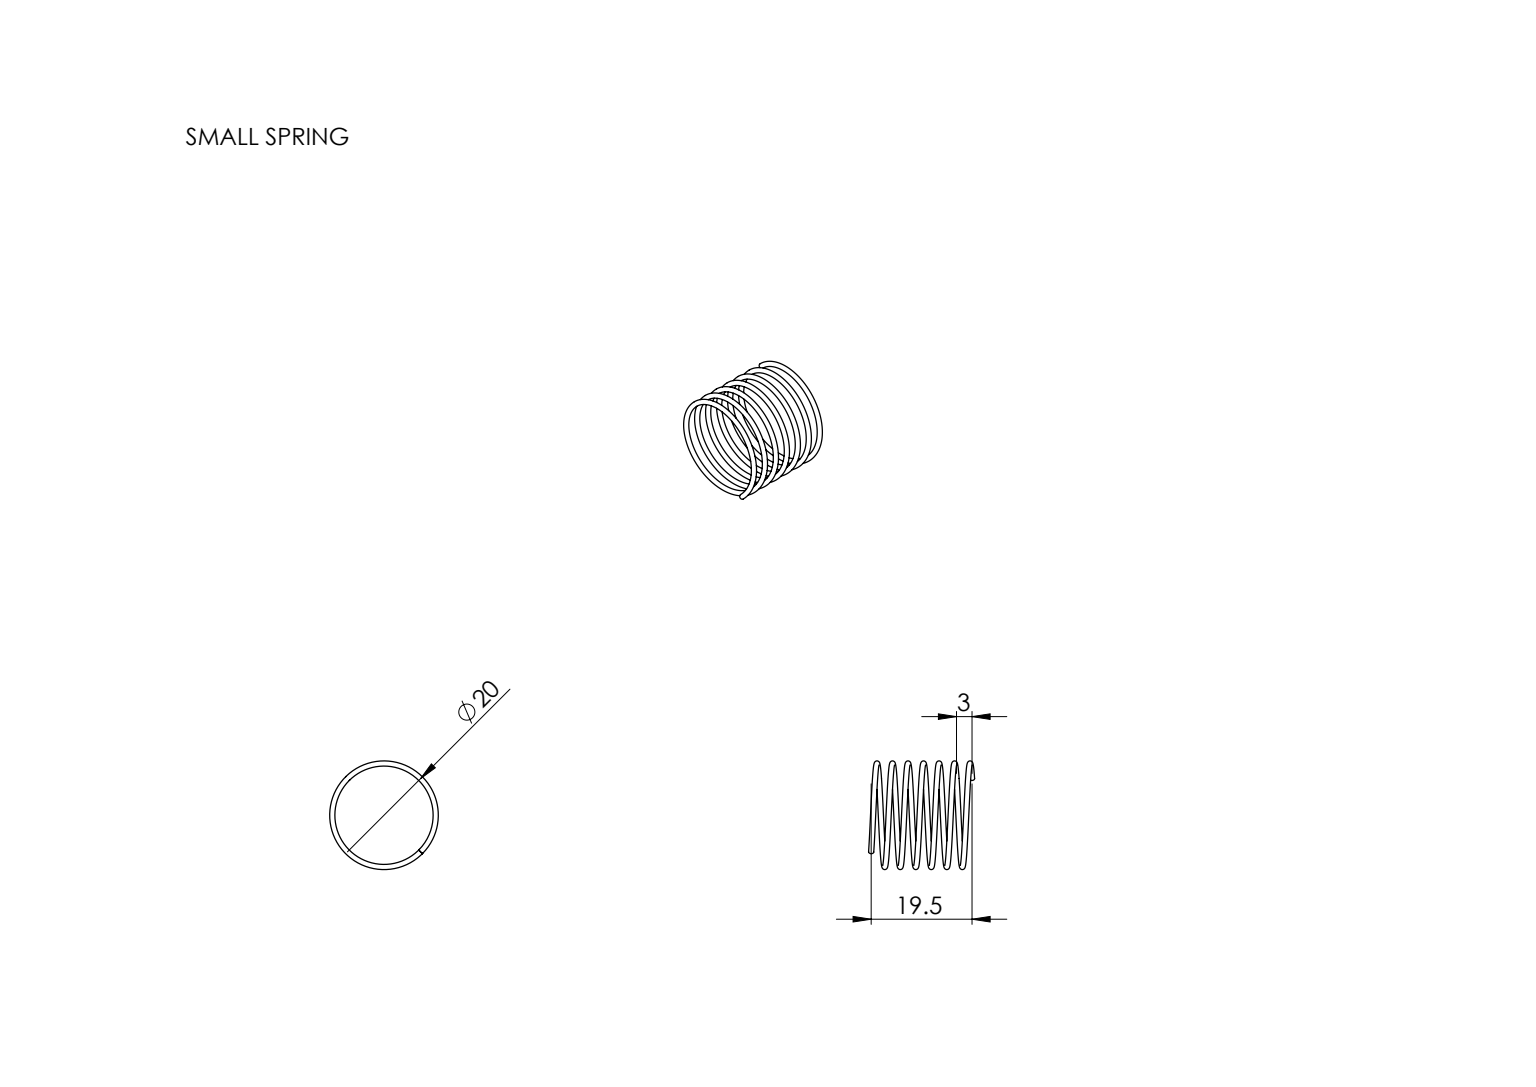
ISO-10303-21;
HEADER;
FILE_DESCRIPTION (('STEP AP214'),
    '1' );
FILE_NAME ('small spring.step',
    '2026-10-08T13:22:57',
    ( '' ),
    ( '' ),
    'SwSTEP 2.0',
    'SolidWorks 2026',
    '' );
FILE_SCHEMA (( 'AUTOMOTIVE_DESIGN' ));
ENDSEC;

DATA;
#1=CARTESIAN_POINT ( 'NONE',  ( -9.837026868206070418, 5.012215536711416952, 5.849999999999989875 ) ) ;
#6=CARTESIAN_POINT ( 'NONE',  ( 9.377220287599001836, 4.724406229267489543, 5.901137918078571687 ) ) ;
#7=CARTESIAN_POINT ( 'NONE',  ( 8.486213763410640709, 4.270415729527937465, 17.90113791807857524 ) ) ;
#23=CARTESIAN_POINT ( 'NONE',  ( -4.312909747525649706, -8.464561979789507973, 14.10000000000000142 ) ) ;
#24=CARTESIAN_POINT ( 'NONE',  ( 4.534861676072320158, -8.900167166472098046, 4.650000000000026112 ) ) ;
#34=CARTESIAN_POINT ( 'NONE',  ( -7.458344646081709328, 7.390897758835804687, 9.998862081921425116 ) ) ;
#40=CARTESIAN_POINT ( 'NONE',  ( -9.865911304835474738, -1.562606840307925848, 8.549999999999963407 ) ) ;
#41=CARTESIAN_POINT ( 'NONE',  ( 5.012215536711511987, -9.837026868205999364, 13.65000000000003233 ) ) ;
#50=CARTESIAN_POINT ( 'NONE',  ( 10.90442828429183919, 1.727091770866679532, 1.049999999999966738 ) ) ;
#55=CARTESIAN_POINT ( 'NONE',  ( 4.766900247265192903, 9.355568503977902850, 12.59999999999999964 ) ) ;
#60=CARTESIAN_POINT ( 'NONE',  ( 4.809394265263009061, 9.333916720356739916, 8.601137918078563871 ) ) ;
#61=CARTESIAN_POINT ( 'NONE',  ( -9.873755945037078874, -1.513077731353019706, 10.55113791807857204 ) ) ;
#72=CARTESIAN_POINT ( 'NONE',  ( 9.865911304835474738, 1.562606840307950051, 19.04999999999997939 ) ) ;
#73=CARTESIAN_POINT ( 'NONE',  ( 8.900167166472154889, -4.534861676072210912, 7.350000000000000533 ) ) ;
#83=CARTESIAN_POINT ( 'NONE',  ( 4.724406229267374968, 9.377220287599055126, 13.59886208192140167 ) ) ;
#84=CARTESIAN_POINT ( 'NONE',  ( 5.056896391392317724, -9.814260835640977731, 14.64886208192141659 ) ) ;
#90=CARTESIAN_POINT ( 'NONE',  ( -1.486127417882243895, 9.383039235653816590, 15.29999999999997939 ) ) ;
#91=CARTESIAN_POINT ( 'NONE',  ( 1.727091770866550968, 10.90442828429186761, 18.44999999999999218 ) ) ;
#99=CARTESIAN_POINT ( 'NONE',  ( -7.806708723663830618, -7.806708723663906113, 8.250000000000028422 ) ) ;
#102=( LENGTH_UNIT ( ) NAMED_UNIT ( * ) SI_UNIT ( .MILLI., .METRE. ) );
#105=CARTESIAN_POINT ( 'NONE',  ( -5.012215536711508435, 9.837026868206029562, 9.150000000000002132 ) ) ;
#108=CARTESIAN_POINT ( 'NONE',  ( -10.91227292449344155, -1.677562661911748965, 4.551137918078585365 ) ) ;
#109=CARTESIAN_POINT ( 'NONE',  ( 9.375578539472099848, -1.533232399699987702, 15.20113791807854575 ) ) ;
#121=CARTESIAN_POINT ( 'NONE',  ( 1.562606840307832368, 9.865911304835503159, 18.44999999999999218 ) ) ;
#122=CARTESIAN_POINT ( 'NONE',  ( 7.063212654743467489, 7.063212654743559860, 3.749999999999997335 ) ) ;
#125=CARTESIAN_POINT ( 'NONE',  ( 7.063212654743468377, 7.063212654743558083, 0.7499999999999762412 ) ) ;
#134=CARTESIAN_POINT ( 'NONE',  ( -8.442910196168309511, -4.355403765523546689, 6.398862081921404155 ) ) ;
#135=CARTESIAN_POINT ( 'NONE',  ( -5.056896391392315948, 9.814260835640997271, 16.14886208192145389 ) ) ;
#141=CARTESIAN_POINT ( 'NONE',  ( 1.562606840307832146, 9.865911304835508489, 15.44999999999997797 ) ) ;
#142=CARTESIAN_POINT ( 'NONE',  ( -9.333916720356675967, -4.809394265263095214, 12.39886208192140948 ) ) ;
#150=CARTESIAN_POINT ( 'NONE',  ( -4.766900247265192014, -9.355568503977867323, 8.099999999999996092 ) ) ;
#151=CARTESIAN_POINT ( 'NONE',  ( -4.766900247265192014, -9.355568503977867323, 8.099999999999996092 ) ) ;
#156=CARTESIAN_POINT ( 'NONE',  ( -5.012215536711508435, 9.837026868206020680, 18.15000000000000924 ) ) ;
#159=CARTESIAN_POINT ( 'NONE',  ( -4.967534682030703586, 9.859792900771061852, 17.15113791807853616 ) ) ;
#160=CARTESIAN_POINT ( 'NONE',  ( 4.490180821391514421, -8.922933199037132113, 12.65113791807859123 ) ) ;
#173=CARTESIAN_POINT ( 'NONE',  ( -1.439022436064386845, 9.390499931835535108, 8.301137918078554279 ) ) ;
#174=CARTESIAN_POINT ( 'NONE',  ( 1.486127417882244783, -9.383039235653782839, 7.800000000000029132 ) ) ;
#177=CARTESIAN_POINT ( 'NONE',  ( -4.312909747525649706, -8.464561979789507973, 2.099999999999990763 ) ) ;
#187=( NAMED_UNIT ( * ) PLANE_ANGLE_UNIT ( ) SI_UNIT ( $, .RADIAN. ) );
#190=CARTESIAN_POINT ( 'NONE',  ( -9.390499931835536884, 1.439022436064298249, 6.698862081921455491 ) ) ;
#191=CARTESIAN_POINT ( 'NONE',  ( -1.533232399700100057, 9.375578539472094519, 1.298862081921425604 ) ) ;
#199=CARTESIAN_POINT ( 'NONE',  ( -4.534861676072319270, 8.900167166472117586, 18.15000000000000924 ) ) ;
#200=CARTESIAN_POINT ( 'NONE',  ( -9.333916720356675967, -4.809394265263096990, 9.398862081921446787 ) ) ;
#206=MANIFOLD_SOLID_BREP ( 'Sweep1', #9455 ) ;
#209=CARTESIAN_POINT ( 'NONE',  ( -10.37072757624895836, 1.642561882922381145, 5.700000000000038369 ) ) ;
#210=CARTESIAN_POINT ( 'NONE',  ( 5.012215536711511987, -9.837026868205999364, 13.65000000000003233 ) ) ;
#213=CARTESIAN_POINT ( 'NONE',  ( 1.727091770866551412, 10.90442828429187117, 15.44999999999997797 ) ) ;
#216=CARTESIAN_POINT ( 'NONE',  ( 9.377220287599001836, 4.724406229267489543, 14.90113791807857879 ) ) ;
#217=CARTESIAN_POINT ( 'NONE',  ( -8.877401133907129704, 4.579542530753042406, 13.85113791807855321 ) ) ;
#226=CARTESIAN_POINT ( 'NONE',  ( 7.098671581784200768, 7.027753727702831021, 8.751137918078539357 ) ) ;
#227=CARTESIAN_POINT ( 'NONE',  ( -8.464561979789474222, -4.312909747525729642, 8.399999999999963052 ) ) ;
#238=( NAMED_UNIT ( * ) SI_UNIT ( $, .STERADIAN. ) SOLID_ANGLE_UNIT ( ) );
#240=CARTESIAN_POINT ( 'NONE',  ( 8.922933199037192509, -4.490180821391404287, 14.34886208192142831 ) ) ;
#242=CARTESIAN_POINT ( 'NONE',  ( -10.89658364409024749, -1.776620879821561694, 15.54886208192143293 ) ) ;
#245=CARTESIAN_POINT ( 'NONE',  ( 0.000000000000000000, 0.000000000000000000, 0.000000000000000000 ) ) ;
#249=CARTESIAN_POINT ( 'NONE',  ( 4.724406229267374968, 9.377220287599060455, 10.59886208192144075 ) ) ;
#258=CARTESIAN_POINT ( 'NONE',  ( 10.90442828429183919, 1.727091770866679532, 10.05000000000002736 ) ) ;
#259=CARTESIAN_POINT ( 'NONE',  ( -10.90442828429183919, -1.727091770866654663, 14.55000000000000249 ) ) ;
#263=CARTESIAN_POINT ( 'NONE',  ( -9.837026868206070418, 5.012215536711416952, 11.84999999999997478 ) ) ;
#266=CARTESIAN_POINT ( 'NONE',  ( 7.390897758835871301, -7.458344646081617846, 18.50113791807859087 ) ) ;
#267=CARTESIAN_POINT ( 'NONE',  ( 9.814260835641038128, -5.056896391392200485, 6.351137918078572753 ) ) ;
#272=CARTESIAN_POINT ( 'NONE',  ( -10.90442828429183919, -1.727091770866655329, 8.549999999999963407 ) ) ;
#278=CARTESIAN_POINT ( 'NONE',  ( 8.486213763410640709, 4.270415729527937465, 5.901137918078571687 ) ) ;
#279=CARTESIAN_POINT ( 'NONE',  ( -4.534861676072319270, 8.900167166472117586, 18.15000000000000924 ) ) ;
#292=CARTESIAN_POINT ( 'NONE',  ( -8.442910196168309511, -4.355403765523546689, 18.39886208192140771 ) ) ;
#293=CARTESIAN_POINT ( 'NONE',  ( 10.89658364409024749, 1.776620879821585897, 20.04886208192142050 ) ) ;
#300=CARTESIAN_POINT ( 'NONE',  ( 4.312909747525650594, 8.464561979789532842, 15.60000000000000320 ) ) ;
#301=CARTESIAN_POINT ( 'NONE',  ( 1.689666864740335894, -10.36326688006721497, 11.79886208192143471 ) ) ;
#307=CARTESIAN_POINT ( 'NONE',  ( 1.642561882922480621, -10.37072757624891750, 7.800000000000029132 ) ) ;
#316=CARTESIAN_POINT ( 'NONE',  ( -5.012215536711506658, 9.837026868206027785, 0.1499999999999952482 ) ) ;
#317=CARTESIAN_POINT ( 'NONE',  ( 7.842167650704563897, 7.771249796623202144, 8.751137918078539357 ) ) ;
#319=CARTESIAN_POINT ( 'NONE',  ( 1.727091770866550968, 10.90442828429187294, 3.450000000000006839 ) ) ;
#327=CARTESIAN_POINT ( 'NONE',  ( 8.877401133907127928, -4.579542530753017537, 9.351137918078563871 ) ) ;
#328=CARTESIAN_POINT ( 'NONE',  ( 8.464561979789474222, 4.312909747525755400, 18.90000000000002700 ) ) ;
#330=( BOUNDED_CURVE ( )  B_SPLINE_CURVE ( 2, ( #1514, #9215, #5487, #10036, #7667, #6246, #5333, #2234, #7861, #8431, #2948, #2187, #6092, #786, #3003, #6917, #1413, #3937, #8645, #6864, #4564, #3053, #741, #637, #9270, #3888, #10090, #7717, #2284, #1567, #6978, #5381, #8538, #4713, #7080, #3840, #3106, #6146, #10139, #1, #1463, #8488, #7032, #7766, #692, #1358, #583, #3729, #6197, #9372, #5429, #8589, #4663, #2129, #7814, #3158, #5271, #4512, #3992, #5682, #3258, #105, #8116, #4813, #4914, #7237, #6452, #5534, #6297, #8061, #7909, #3313, #4967, #989, #9631, #2434, #8693, #8897, #4042, #263, #9481, #942, #8852, #7290, #55, #6399, #1719, #4140, #3363, #3213, #7963, #836, #1045, #2534, #5579, #9576, #6498, #1811, #4190, #4763, #7340, #1665, #1762, #213, #7188, #894, #9677, #2480, #5634, #2585, #8800, #8742, #2384, #5730, #1614, #7138, #6349, #4864, #9527, #8010, #4087, #156, #8365, #9874, #1287, #9727, #9156, #7438, #2013, #5168, #7593 ),
 .UNSPECIFIED., .F., .T. ) 
 B_SPLINE_CURVE_WITH_KNOTS ( ( 3, 2, 2, 2, 2, 2, 2, 2, 2, 2, 2, 2, 2, 2, 2, 2, 2, 2, 2, 2, 2, 2, 2, 2, 2, 2, 2, 2, 2, 2, 2, 2, 2, 2, 2, 2, 2, 2, 2, 2, 2, 2, 2, 2, 2, 2, 2, 2, 2, 2, 2, 2, 2, 2, 2, 2, 2, 2, 2, 2, 2, 2, 2, 2, 2, 3 ),
 ( 0.000000000000000000, 0.01428571428571428527, 0.02857142857142857054, 0.04285714285714285060, 0.05714285714285714107, 0.07142857142857142461, 0.08571428571428570120, 0.1000000000000000056, 0.1142857142857142821, 0.1285714285714285587, 0.1428571428571428492, 0.1571428571428571397, 0.1714285714285714024, 0.1857142857142857206, 0.2000000000000000111, 0.2142857142857142738, 0.2285714285714285643, 0.2428571428571428548, 0.2571428571428571175, 0.2714285714285714080, 0.2857142857142856984, 0.2999999999999999889, 0.3142857142857142794, 0.3285714285714285698, 0.3428571428571428048, 0.3571428571428571508, 0.3714285714285714413, 0.3857142857142857317, 0.4000000000000000222, 0.4142857142857143127, 0.4285714285714285476, 0.4428571428571428381, 0.4571428571428571286, 0.4714285714285714191, 0.4857142857142857095, 0.5000000000000000000, 0.5142857142857142350, 0.5285714285714285809, 0.5428571428571428159, 0.5571428571428571619, 0.5714285714285713969, 0.5857142857142857428, 0.5999999999999999778, 0.6142857142857143238, 0.6285714285714285587, 0.6428571428571429047, 0.6571428571428571397, 0.6714285714285713746, 0.6857142857142856096, 0.6999999999999999556, 0.7142857142857143016, 0.7285714285714285365, 0.7428571428571428825, 0.7571428571428571175, 0.7714285714285714635, 0.7857142857142856984, 0.8000000000000000444, 0.8142857142857143904, 0.8285714285714286254, 0.8428571428571428603, 0.8571428571428570953, 0.8714285714285714413, 0.8857142857142856762, 0.9000000000000000222, 0.9142857142857142572, 0.9285714285714286031 ),
 .UNSPECIFIED. ) 
 CURVE ( )  GEOMETRIC_REPRESENTATION_ITEM ( )  RATIONAL_B_SPLINE_CURVE ( ( 1.000000000000000000, 0.9510565162951535312, 1.000000000000000000, 0.9510565162951535312, 1.000000000000000000, 0.9510565162951535312, 1.000000000000000000, 0.9510565162951535312, 1.000000000000000000, 0.9510565162951535312, 1.000000000000000000, 0.9510565162951535312, 1.000000000000000000, 0.9510565162951535312, 1.000000000000000000, 0.9510565162951535312, 1.000000000000000000, 0.9510565162951535312, 1.000000000000000000, 0.9510565162951535312, 1.000000000000000000, 0.9510565162951535312, 1.000000000000000000, 0.9510565162951535312, 1.000000000000000000, 0.9510565162951535312, 1.000000000000000000, 0.9510565162951535312, 1.000000000000000000, 0.9510565162951535312, 1.000000000000000000, 0.9510565162951535312, 1.000000000000000000, 0.9510565162951535312, 1.000000000000000000, 0.9510565162951535312, 1.000000000000000000, 0.9510565162951535312, 1.000000000000000000, 0.9510565162951535312, 1.000000000000000000, 0.9510565162951535312, 1.000000000000000000, 0.9510565162951535312, 1.000000000000000000, 0.9510565162951535312, 1.000000000000000000, 0.9510565162951535312, 1.000000000000000000, 0.9510565162951535312, 1.000000000000000000, 0.9510565162951535312, 1.000000000000000000, 0.9510565162951535312, 1.000000000000000000, 0.9510565162951535312, 1.000000000000000000, 0.9510565162951535312, 1.000000000000000000, 0.9510565162951535312, 1.000000000000000000, 0.9510565162951535312, 1.000000000000000000, 0.9510565162951535312, 1.000000000000000000, 0.9510565162951535312, 1.000000000000000000, 0.9510565162951535312, 1.000000000000000000, 0.9510565162951535312, 1.000000000000000000, 0.9510565162951535312, 1.000000000000000000, 0.9510565162951535312, 1.000000000000000000, 0.9510565162951535312, 1.000000000000000000, 0.9510565162951535312, 1.000000000000000000, 0.9510565162951535312, 1.000000000000000000, 0.9510565162951535312, 1.000000000000000000, 0.9510565162951535312, 1.000000000000000000, 0.9510565162951535312, 1.000000000000000000, 0.9510565162951535312, 1.000000000000000000, 0.9510565162951535312, 1.000000000000000000, 0.9510565162951535312, 1.000000000000000000, 0.9510565162951535312, 1.000000000000000000, 0.9510565162951535312, 1.000000000000000000, 0.9510565162951535312, 1.000000000000000000, 0.9510565162951535312, 1.000000000000000000, 0.9510565162951535312, 1.000000000000000000, 0.9510565162951535312, 1.000000000000000000, 0.9510565162951535312, 1.000000000000000000, 0.9510565162951535312, 1.000000000000000000, 0.9510565162951535312, 1.000000000000000000, 0.9510565162951535312, 1.000000000000000000, 0.9510565162951535312, 1.000000000000000000, 0.9510565162951535312, 1.000000000000000000, 0.9510565162951535312, 1.000000000000000000, 0.9510565162951535312, 1.000000000000000000, 0.9510565162951535312, 1.000000000000000000, 0.9510565162951535312, 1.000000000000000000, 0.9510565162951535312, 1.000000000000000000, 0.9510565162951535312, 1.000000000000000000, 0.9510565162951535312, 1.000000000000000000 ) ) 
 REPRESENTATION_ITEM ( '' )  );
#342=CARTESIAN_POINT ( 'NONE',  ( -4.270415729527831772, -8.486213763410670907, 15.09886208192144430 ) ) ;
#343=CARTESIAN_POINT ( 'NONE',  ( 9.390499931835536884, -1.439022436064273158, 8.198862081921454603 ) ) ;
#353=CARTESIAN_POINT ( 'NONE',  ( -4.724406229267374968, -9.377220287599040915, 9.098862081921437195 ) ) ;
#361=CARTESIAN_POINT ( 'NONE',  ( 7.424621202458790314, -7.424621202458697944, 16.50000000000001421 ) ) ;
#367=CARTESIAN_POINT ( 'NONE',  ( -7.027753727702738651, -7.098671581784268270, 3.248862081921429112 ) ) ;
#370=CARTESIAN_POINT ( 'NONE',  ( 7.390897758835871301, -7.458344646081617846, 15.50113791807859620 ) ) ;
#371=CARTESIAN_POINT ( 'NONE',  ( -1.776620879821455556, -10.89658364409025637, 0.9511379180785689558 ) ) ;
#376=CARTESIAN_POINT ( 'NONE',  ( 9.837026868206066865, -5.012215536711392083, 7.350000000000000533 ) ) ;
#381=CARTESIAN_POINT ( 'NONE',  ( -9.375578539472099848, 1.533232399700011461, 4.701137918078535982 ) ) ;
#382=CARTESIAN_POINT ( 'NONE',  ( -6.717514421272238856, 6.717514421272181124, 12.00000000000001066 ) ) ;
#392=FILL_AREA_STYLE ('',( #2563 ) ) ;
#396=CARTESIAN_POINT ( 'NONE',  ( 8.442910196168311288, 4.355403765523576887, 16.89886208192141126 ) ) ;
#397=CARTESIAN_POINT ( 'NONE',  ( -8.922933199037192509, 4.490180821391428267, 3.848862081921410105 ) ) ;
#411=CARTESIAN_POINT ( 'NONE',  ( -10.37072757624895836, 1.642561882922380923, 17.69999999999999218 ) ) ;
#418=CARTESIAN_POINT ( 'NONE',  ( 6.751237864895159646, -6.683790977649233689, 5.498862081921462419 ) ) ;
#420=CARTESIAN_POINT ( 'NONE',  ( -10.90442828429183919, -1.727091770866655329, 5.549999999999999822 ) ) ;
#421=CARTESIAN_POINT ( 'NONE',  ( -10.91227292449344155, -1.677562661911748965, 4.551137918078585365 ) ) ;
#424=CARTESIAN_POINT ( 'NONE',  ( 4.766900247265192903, 9.355568503977911732, 9.599999999999997868 ) ) ;
#431=CARTESIAN_POINT ( 'NONE',  ( -6.683790977649319842, 6.751237864895094809, 14.00113791807859620 ) ) ;
#432=CARTESIAN_POINT ( 'NONE',  ( 9.873755945037075321, 1.513077731353043909, 0.05113791807855379290 ) ) ;
#444=CARTESIAN_POINT ( 'NONE',  ( 1.513077731352925115, 9.873755945037103743, 16.44886208192140131 ) ) ;
#445=CARTESIAN_POINT ( 'NONE',  ( 9.858066664633883036, 1.612135949262857082, 11.04886208192144359 ) ) ;
#446=CARTESIAN_POINT ( 'NONE',  ( -5.012215536711506658, 9.837026868206027785, 15.14999999999998259 ) ) ;
#462=CARTESIAN_POINT ( 'NONE',  ( -5.056896391392315948, 9.814260835640997271, 1.148862081921408151 ) ) ;
#463=SHAPE_DEFINITION_REPRESENTATION ( #3602, #1843 ) ;
#469=CARTESIAN_POINT ( 'NONE',  ( -8.442910196168309511, -4.355403765523544024, 3.398862081921444123 ) ) ;
#470=CARTESIAN_POINT ( 'NONE',  ( -4.766900247265192014, -9.355568503977867323, 8.099999999999996092 ) ) ;
#471=CARTESIAN_POINT ( 'NONE',  ( -10.91227292449344155, -1.677562661911748965, 7.551137918078578259 ) ) ;
#473=CARTESIAN_POINT ( 'NONE',  ( -1.642561882922479732, 10.37072757624895303, 3.299999999999969624 ) ) ;
#479=CARTESIAN_POINT ( 'NONE',  ( -9.375578539472099848, 1.533232399700011461, 13.70113791807854398 ) ) ;
#480=CARTESIAN_POINT ( 'NONE',  ( 7.063212654743467489, 7.063212654743559860, 18.74999999999998934 ) ) ;
#491=CARTESIAN_POINT ( 'NONE',  ( -7.806708723663830618, -7.806708723663906113, 2.249999999999986233 ) ) ;
#492=CARTESIAN_POINT ( 'NONE',  ( -9.865911304835474738, -1.562606840307925626, 5.549999999999999822 ) ) ;
#493=CARTESIAN_POINT ( 'NONE',  ( 9.858066664633883036, 1.612135949262857082, 8.048862081921450695 ) ) ;
#495=CARTESIAN_POINT ( 'NONE',  ( -4.766900247265192014, -9.355568503977876205, 17.10000000000000497 ) ) ;
#504=CARTESIAN_POINT ( 'NONE',  ( 7.424621202458790314, -7.424621202458697944, 16.50000000000001421 ) ) ;
#510=CARTESIAN_POINT ( 'NONE',  ( -10.90442828429183919, -1.727091770866654663, 14.55000000000000249 ) ) ;
#518=DIRECTION ( 'NONE',  ( 0.7063021515967569108, 0.7063021515967620179, -0.04769215134145658730 ) ) ;
#521=CARTESIAN_POINT ( 'NONE',  ( 9.858066664633883036, 1.612135949262857526, 5.048862081921459577 ) ) ;
#523=CARTESIAN_POINT ( 'NONE',  ( 1.727091770866550968, 10.90442828429186761, 6.449999999999969091 ) ) ;
#524=CARTESIAN_POINT ( 'NONE',  ( -10.36326688006724162, 1.689666864740236640, 13.70113791807854398 ) ) ;
#527=CARTESIAN_POINT ( 'NONE',  ( -7.806708723663830618, -7.806708723663902560, 14.25000000000001243 ) ) ;
#534=CARTESIAN_POINT ( 'NONE',  ( -4.355403765523468529, -8.442910196168352144, 13.10113791807856920 ) ) ;
#535=CARTESIAN_POINT ( 'NONE',  ( -9.375578539472099848, 1.533232399700010351, 7.701137918078540423 ) ) ;
#546=CARTESIAN_POINT ( 'NONE',  ( 1.727091770866550968, 10.90442828429187294, 0.4499999999999856337 ) ) ;
#547=CARTESIAN_POINT ( 'NONE',  ( 6.717514421272239744, -6.717514421272154479, 4.500000000000003553 ) ) ;
#548=CARTESIAN_POINT ( 'NONE',  ( 8.442910196168311288, 4.355403765523574222, 13.89886208192141126 ) ) ;
#550=CARTESIAN_POINT ( 'NONE',  ( 7.806708723663831506, 7.806708723663930982, 12.75000000000000533 ) ) ;
#558=CARTESIAN_POINT ( 'NONE',  ( 9.355568503977840678, 4.766900247265305701, 18.90000000000002700 ) ) ;
#563=CARTESIAN_POINT ( 'NONE',  ( -1.642561882922479732, 10.37072757624895303, 18.29999999999998295 ) ) ;
#575=CARTESIAN_POINT ( 'NONE',  ( -4.579542530753125895, 8.877401133907090625, 1.148862081921408151 ) ) ;
#577=CARTESIAN_POINT ( 'NONE',  ( 9.355568503977840678, 4.766900247265305701, 6.899999999999961275 ) ) ;
#578=CARTESIAN_POINT ( 'NONE',  ( 1.776620879821457333, 10.89658364409028124, 17.45113791807857240 ) ) ;
#581=CARTESIAN_POINT ( 'NONE',  ( 9.837026868206066865, -5.012215536711392083, 19.34999999999996945 ) ) ;
#583=CARTESIAN_POINT ( 'NONE',  ( 9.355568503977840678, 4.766900247265305701, 6.899999999999961275 ) ) ;
#588=CARTESIAN_POINT ( 'NONE',  ( -6.683790977649319842, 6.751237864895094809, 11.00113791807855002 ) ) ;
#589=CARTESIAN_POINT ( 'NONE',  ( -7.098671581784199880, -7.027753727702809705, 4.251137918078595312 ) ) ;
#601=CARTESIAN_POINT ( 'NONE',  ( 1.486127417882244783, -9.383039235653782839, 10.80000000000003268 ) ) ;
#602=CARTESIAN_POINT ( 'NONE',  ( 9.390499931835536884, -1.439022436064272936, 17.19886208192146171 ) ) ;
#613=CARTESIAN_POINT ( 'NONE',  ( -7.424621202458789426, 7.424621202458724589, 18.00000000000001421 ) ) ;
#617=CARTESIAN_POINT ( 'NONE',  ( -7.771249796623103556, -7.842167650704634063, 6.248862081921465084 ) ) ;
#629=CARTESIAN_POINT ( 'NONE',  ( -1.533232399700100057, 9.375578539472098072, 7.298862081921430267 ) ) ;
#631=CARTESIAN_POINT ( 'NONE',  ( 10.90442828429183919, 1.727091770866678422, 4.049999999999988276 ) ) ;
#632=CARTESIAN_POINT ( 'NONE',  ( -7.390897758835869524, 7.458344646081637386, 11.00113791807855002 ) ) ;
#637=CARTESIAN_POINT ( 'NONE',  ( 1.727091770866551412, 10.90442828429187117, 3.450000000000007283 ) ) ;
#642=CARTESIAN_POINT ( 'NONE',  ( -9.375578539472099848, 1.533232399700011683, 10.70113791807854220 ) ) ;
#643=CARTESIAN_POINT ( 'NONE',  ( 4.490180821391514421, -8.922933199037132113, 9.651137918078598332 ) ) ;
#654=CARTESIAN_POINT ( 'NONE',  ( 9.865911304835474738, 1.562606840307950051, 10.05000000000002736 ) ) ;
#655=CARTESIAN_POINT ( 'NONE',  ( 4.270415729527831772, 8.486213763410688671, 13.59886208192144430 ) ) ;
#663=CARTESIAN_POINT ( 'NONE',  ( 4.766900247265192903, 9.355568503977902850, 18.60000000000000497 ) ) ;
#667=CARTESIAN_POINT ( 'NONE',  ( -9.333916720356675967, -4.809394265263096990, 6.398862081921446787 ) ) ;
#672=CARTESIAN_POINT ( 'NONE',  ( -9.865911304835474738, -1.562606840307925626, 11.54999999999998295 ) ) ;
#681=CARTESIAN_POINT ( 'NONE',  ( -4.579542530753125895, 8.877401133907090625, 7.148862081921437017 ) ) ;
#684=CARTESIAN_POINT ( 'NONE',  ( 1.595456901104624459, -10.37818827243065201, 12.80113791807860224 ) ) ;
#692=CARTESIAN_POINT ( 'NONE',  ( 4.766900247265192903, 9.355568503977911732, 6.599999999999994316 ) ) ;
#697=CARTESIAN_POINT ( 'NONE',  ( -7.390897758835869524, 7.458344646081644491, 8.001137918078546463 ) ) ;
#698=CARTESIAN_POINT ( 'NONE',  ( 9.873755945037075321, 1.513077731353043243, 3.051137918078546285 ) ) ;
#708=CARTESIAN_POINT ( 'NONE',  ( 6.717514421272239744, -6.717514421272154479, 7.500000000000007105 ) ) ;
#709=CARTESIAN_POINT ( 'NONE',  ( -6.717514421272238856, 6.717514421272181124, 0.000000000000000000 ) ) ;
#717=CARTESIAN_POINT ( 'NONE',  ( 10.37072757624895836, -1.642561882922356498, 16.19999999999999218 ) ) ;
#720=CARTESIAN_POINT ( 'NONE',  ( 7.771249796623105333, 7.842167650704658932, 10.74886208192140913 ) ) ;
#725=CARTESIAN_POINT ( 'NONE',  ( 9.383039235653818366, -1.486127417882129986, 7.199999999999984190 ) ) ;
#732=CARTESIAN_POINT ( 'NONE',  ( -4.579542530753125895, 8.877401133907083519, 13.14886208192146633 ) ) ;
#734=CARTESIAN_POINT ( 'NONE',  ( 4.766900247265192903, 9.355568503977902850, 0.5999999999999894307 ) ) ;
#735=CARTESIAN_POINT ( 'NONE',  ( -7.806708723663830618, -7.806708723663901672, 5.250000000000008882 ) ) ;
#741=CARTESIAN_POINT ( 'NONE',  ( -1.642561882922479732, 10.37072757624895303, 3.299999999999969624 ) ) ;
#744=CARTESIAN_POINT ( 'NONE',  ( -1.776620879821455556, -10.89658364409025637, 9.951137918078590161 ) ) ;
#745=CARTESIAN_POINT ( 'NONE',  ( 6.683790977649321619, -6.751237864895082375, 3.501137918078585987 ) ) ;
#756=CARTESIAN_POINT ( 'NONE',  ( 8.486213763410640709, 4.270415729527937465, -0.09886208192143307316 ) ) ;
#757=CARTESIAN_POINT ( 'NONE',  ( 9.858066664633883036, 1.612135949262858858, 14.04886208192143471 ) ) ;
#766=CARTESIAN_POINT ( 'NONE',  ( -10.89658364409024749, -1.776620879821561472, 9.548862081921404510 ) ) ;
#771=CARTESIAN_POINT ( 'NONE',  ( 1.486127417882244783, -9.383039235653782839, 7.800000000000029132 ) ) ;
#772=CARTESIAN_POINT ( 'NONE',  ( 4.724406229267374968, 9.377220287599055126, 1.598862081921434308 ) ) ;
#774=ORIENTED_EDGE ( 'NONE', *, *, #1414, .F. ) ;
#779=CARTESIAN_POINT ( 'NONE',  ( -5.012215536711506658, 9.837026868206027785, 3.149999999999957723 ) ) ;
#780=CARTESIAN_POINT ( 'NONE',  ( 4.766900247265192903, 9.355568503977911732, 6.599999999999994316 ) ) ;
#786=CARTESIAN_POINT ( 'NONE',  ( -1.727091770866549414, -10.90442828429184807, 1.949999999999996403 ) ) ;
#790=CARTESIAN_POINT ( 'NONE',  ( 4.967534682030706250, -9.859792900771042312, 3.651137918078570355 ) ) ;
#791=CARTESIAN_POINT ( 'NONE',  ( -7.098671581784199880, -7.027753727702809705, 13.25113791807857311 ) ) ;
#802=CARTESIAN_POINT ( 'NONE',  ( 7.063212654743467489, 7.063212654743557195, 12.75000000000000533 ) ) ;
#803=CARTESIAN_POINT ( 'NONE',  ( 8.464561979789474222, 4.312909747525755400, 6.899999999999961275 ) ) ;
#806=CARTESIAN_POINT ( 'NONE',  ( 1.562606840307832146, 9.865911304835508489, 3.450000000000007283 ) ) ;
#814=CARTESIAN_POINT ( 'NONE',  ( -10.89658364409024749, -1.776620879821559917, 6.548862081921412504 ) ) ;
#819=CARTESIAN_POINT ( 'NONE',  ( 4.312909747525650594, 8.464561979789532842, 12.59999999999999964 ) ) ;
#820=CARTESIAN_POINT ( 'NONE',  ( -10.90442828429183919, -1.727091770866654663, 17.55000000000002913 ) ) ;
#828=CARTESIAN_POINT ( 'NONE',  ( -7.424621202458789426, 7.424621202458724589, 0.000000000000000000 ) ) ;
#829=CARTESIAN_POINT ( 'NONE',  ( -7.806708723663830618, -7.806708723663906113, 2.249999999999986233 ) ) ;
#836=CARTESIAN_POINT ( 'NONE',  ( 5.012215536711512875, -9.837026868206002916, 13.65000000000003411 ) ) ;
#839=CARTESIAN_POINT ( 'NONE',  ( -9.814260835641038128, 5.056896391392221801, 7.851137918078569200 ) ) ;
#840=CARTESIAN_POINT ( 'NONE',  ( -4.490180821391513533, 8.922933199037158758, 11.15113791807855215 ) ) ;
#855=CARTESIAN_POINT ( 'NONE',  ( 9.383039235653818366, -1.486127417882131097, 13.19999999999998863 ) ) ;
#856=CARTESIAN_POINT ( 'NONE',  ( -9.865911304835474738, -1.562606840307925626, 2.550000000000035350 ) ) ;
#859=CARTESIAN_POINT ( 'NONE',  ( 4.534861676072321046, -8.900167166472098046, 1.650000000000006128 ) ) ;
#869=CARTESIAN_POINT ( 'NONE',  ( 10.89658364409024749, 1.776620879821587229, 14.04886208192143471 ) ) ;
#870=CARTESIAN_POINT ( 'NONE',  ( -9.333916720356675967, -4.809394265263096990, 15.39886208192141126 ) ) ;
#877=CARTESIAN_POINT ( 'NONE',  ( 7.063212654743468377, 7.063212654743554531, 9.749999999999982236 ) ) ;
#878=CARTESIAN_POINT ( 'NONE',  ( 10.37072757624895836, -1.642561882922356498, 13.19999999999998863 ) ) ;
#879=VERTEX_POINT ( 'NONE', #8076 ) ;
#888=CARTESIAN_POINT ( 'NONE',  ( -5.012215536711506658, 9.837026868206022456, 6.149999999999980815 ) ) ;
#891=SURFACE_STYLE_USAGE ( .BOTH. , #7906 ) ;
#894=CARTESIAN_POINT ( 'NONE',  ( 7.806708723663832394, 7.806708723663926541, 15.74999999999996803 ) ) ;
#897=CARTESIAN_POINT ( 'NONE',  ( -10.36326688006724162, 1.689666864740236640, 4.701137918078535982 ) ) ;
#898=CARTESIAN_POINT ( 'NONE',  ( -6.683790977649319842, 6.751237864895094809, 14.00113791807859620 ) ) ;
#907=CARTESIAN_POINT ( 'NONE',  ( -1.486127417882243895, 9.383039235653816590, 18.29999999999998295 ) ) ;
#908=CARTESIAN_POINT ( 'NONE',  ( 1.562606840307832368, 9.865911304835510265, 3.450000000000006839 ) ) ;
#911=CARTESIAN_POINT ( 'NONE',  ( 4.312909747525650594, 8.464561979789532842, 3.599999999999992095 ) ) ;
#918=CARTESIAN_POINT ( 'NONE',  ( -7.027753727702738651, -7.098671581784262941, 6.248862081921465084 ) ) ;
#919=CARTESIAN_POINT ( 'NONE',  ( -9.333916720356675967, -4.809394265263096990, 15.39886208192141126 ) ) ;
#927=CARTESIAN_POINT ( 'NONE',  ( -7.771249796623103556, -7.842167650704634063, 12.24886208192144998 ) ) ;
#935=CARTESIAN_POINT ( 'NONE',  ( 1.727091770866550968, 10.90442828429187294, 12.44999999999995666 ) ) ;
#936=CARTESIAN_POINT ( 'NONE',  ( -5.012215536711506658, 9.837026868206027785, 9.150000000000003908 ) ) ;
#938=( NAMED_UNIT ( * ) SI_UNIT ( $, .STERADIAN. ) SOLID_ANGLE_UNIT ( ) );
#942=CARTESIAN_POINT ( 'NONE',  ( -5.012215536711508435, 9.837026868206027785, 12.14999999999996483 ) ) ;
#946=CARTESIAN_POINT ( 'NONE',  ( -4.809394265263009061, -9.333916720356718599, 10.10113791807856742 ) ) ;
#947=CARTESIAN_POINT ( 'NONE',  ( -8.486213763410637156, -4.270415729527911708, 16.40113791807857524 ) ) ;
#956=CARTESIAN_POINT ( 'NONE',  ( -4.490180821391513533, 8.922933199037158758, -0.8488620819214613977 ) ) ;
#957=CARTESIAN_POINT ( 'NONE',  ( 1.562606840307832368, 9.865911304835503159, 6.449999999999969091 ) ) ;
#960=CARTESIAN_POINT ( 'NONE',  ( 9.865911304835478290, 1.562606840307950273, 1.049999999999966738 ) ) ;
#966=SURFACE_STYLE_USAGE ( .BOTH. , #8087 ) ;
#967=EDGE_CURVE ( 'NONE', #1139, #7327, #8083, .T. ) ;
#968=CARTESIAN_POINT ( 'NONE',  ( 9.390499931835536884, -1.439022436064272270, 11.19886208192145816 ) ) ;
#969=CARTESIAN_POINT ( 'NONE',  ( -5.056896391392315948, 9.814260835640997271, 19.14886208192144679 ) ) ;
#976=CARTESIAN_POINT ( 'NONE',  ( -9.383039235653820143, 1.486127417882154411, 14.69999999999999041 ) ) ;
#977=CARTESIAN_POINT ( 'NONE',  ( 7.771249796623105333, 7.842167650704658932, 7.748862081921418010 ) ) ;
#984=CARTESIAN_POINT ( 'NONE',  ( -9.355568503977838901, -4.766900247265280832, 8.399999999999963052 ) ) ;
#985=CARTESIAN_POINT ( 'NONE',  ( -1.727091770866549414, -10.90442828429184630, 10.95000000000000462 ) ) ;
#989=CARTESIAN_POINT ( 'NONE',  ( -1.727091770866549414, -10.90442828429184807, 10.95000000000000284 ) ) ;
#993=CARTESIAN_POINT ( 'NONE',  ( 7.842167650704563897, 7.771249796623202144, 17.75113791807856245 ) ) ;
#994=CARTESIAN_POINT ( 'NONE',  ( -4.490180821391513533, 8.922933199037153429, 14.15113791807854327 ) ) ;
#1007=CARTESIAN_POINT ( 'NONE',  ( 1.439022436064387511, -9.390499931835512015, 9.801137918078557831 ) ) ;
#1008=CARTESIAN_POINT ( 'NONE',  ( -9.383039235653820143, 1.486127417882155299, 2.700000000000035705 ) ) ;
#1019=CARTESIAN_POINT ( 'NONE',  ( 6.717514421272239744, -6.717514421272154479, 1.500000000000001332 ) ) ;
#1020=CARTESIAN_POINT ( 'NONE',  ( 9.858066664633883036, 1.612135949262857526, 2.048862081921423162 ) ) ;
#1030=CARTESIAN_POINT ( 'NONE',  ( 8.464561979789474222, 4.312909747525755400, 18.90000000000002700 ) ) ;
#1031=CARTESIAN_POINT ( 'NONE',  ( 5.056896391392317724, -9.814260835640970626, 5.648862081921440570 ) ) ;
#1040=CARTESIAN_POINT ( 'NONE',  ( -7.424621202458789426, 7.424621202458723701, 9.000000000000007105 ) ) ;
#1041=CARTESIAN_POINT ( 'NONE',  ( 4.766900247265192903, 9.355568503977902850, 18.60000000000000497 ) ) ;
#1045=CARTESIAN_POINT ( 'NONE',  ( 1.642561882922480621, -10.37072757624892638, 13.80000000000003446 ) ) ;
#1050=CARTESIAN_POINT ( 'NONE',  ( 10.36326688006723984, -1.689666864740210883, 18.20113791807854398 ) ) ;
#1051=CARTESIAN_POINT ( 'NONE',  ( 10.36326688006723984, -1.689666864740210883, 9.201137918078538647 ) ) ;
#1062=CARTESIAN_POINT ( 'NONE',  ( -1.439022436064386845, 9.390499931835526226, 2.301137918078551614 ) ) ;
#1063=CARTESIAN_POINT ( 'NONE',  ( -9.383039235653820143, 1.486127417882155299, 17.69999999999999218 ) ) ;
#1074=CARTESIAN_POINT ( 'NONE',  ( 1.533232399700100945, -9.375578539472067874, 17.79886208192143471 ) ) ;
#1075=CARTESIAN_POINT ( 'NONE',  ( 9.333916720356675967, 4.809394265263123636, 13.89886208192141126 ) ) ;
#1076=ADVANCED_FACE ( 'NONE', ( #2329 ), #5267, .T. ) ;
#1083=CARTESIAN_POINT ( 'NONE',  ( -10.37818827243067688, 1.595456901104523428, 9.698862081921454603 ) ) ;
#1089=CARTESIAN_POINT ( 'NONE',  ( 10.37072757624895836, -1.642561882922355609, 7.199999999999984190 ) ) ;
#1097=CARTESIAN_POINT ( 'NONE',  ( -4.809394265263009061, -9.333916720356716823, 16.10113791807856742 ) ) ;
#1098=CARTESIAN_POINT ( 'NONE',  ( 10.91227292449344155, 1.677562661911773390, 3.051137918078546285 ) ) ;
#1103=CARTESIAN_POINT ( 'NONE',  ( -9.355568503977838901, -4.766900247265279944, 11.39999999999996660 ) ) ;
#1110=CARTESIAN_POINT ( 'NONE',  ( -9.873755945037078874, -1.513077731353019706, 4.551137918078585365 ) ) ;
#1111=CARTESIAN_POINT ( 'NONE',  ( 9.383039235653818366, -1.486127417882131097, 13.19999999999998863 ) ) ;
#1120=CARTESIAN_POINT ( 'NONE',  ( 9.858066664633883036, 1.612135949262857526, 17.04886208192142760 ) ) ;
#1121=CARTESIAN_POINT ( 'NONE',  ( -8.922933199037192509, 4.490180821391428267, 9.848862081921437195 ) ) ;
#1122=( BOUNDED_SURFACE ( )  B_SPLINE_SURFACE ( 3, 2, ( 
 ( #7735, #4471, #7626, #546, #6163, #10051, #2910, #6828, #9339, #1376, #4527, #2963, #6882, #1262, #7570, #491, #3637, #6771, #9184, #2089, #8327, #5123, #473, #319, #8963, #7549, #2693, #5883, #5222, #9062, #5986, #6698, #1970, #1921, #6652, #1245, #4295, #8275, #9167, #6603, #2072, #5935, #9835, #2020, #5835, #9114, #5178, #9790, #5023, #376, #8376, #3615, #1196, #8167, #4400, #4347, #7500, #272, #6750, #3418, #3466, #9938, #2843, #1298, #424, #7349, #9012, #1875, #5069, #6554, #8220, #9737, #3568, #9884, #2639, #5788, #1103, #4245, #2786, #7397, #1147, #7449, #3527, #2738, #3677, #2318, #8787, #7607, #878, #5471, #3199, #41, #9987, #4451, #4510, #527, #5520, #1650, #4797, #1552, #8729, #7951, #2127, #9563, #9213, #2420, #6334, #6862, #7665, #10174, #7895, #4750, #8630, #9408, #4030, #3090, #6231, #820, #4699, #7846, #2467, #7174, #1601, #91, #3246, #7064, #5568, #2368, #6384, #581, #6037 ),
 ( #6281, #5618, #3974, #9466, #772, #3920, #6810, #9555, #8679, #2893, #3727, #5268, #9514, #3137, #8429, #7125, #1355, #9766, #4125, #9619, #4951, #9816, #5051, #3398, #4225, #5002, #2521, #8148, #4274, #9713, #8102, #1031, #1128, #7425, #6533, #8048, #8838, #6582, #4177, #9665, #4075, #2618, #1751, #5763, #3352, #977, #7274, #4900, #5670, #7374, #8991, #3501, #3443, #8196, #353, #6632, #200, #2717, #1083, #7999, #6487, #5861, #7326, #3295, #249, #1704, #4849, #7224, #2573, #8935, #1852, #1902, #301, #6436, #2670, #927, #142, #5815, #5715, #8884, #1797, #3238, #1791, #3391, #83, #4019, #1075, #869, #4170, #4942, #8775, #9554, #1697, #9658, #6478, #7214, #919, #242, #4841, #7992, #2566, #135, #4068, #4215, #2610, #3344, #8924, #4995, #8831, #7318, #4118, #9703, #2460, #7939, #6525, #3286, #4893, #7367, #8040, #8140, #5707, #969, #6428, #5663, #5755, #9610, #7264, #293, #5608, #6325, #8091 ),
 ( #7164, #2514, #191, #1742, #6376, #1841, #8877, #1020, #9507, #2411, #5559, #8719, #1641, #4786, #8394, #9904, #1319, #6573, #2757, #397, #5808, #5197, #7629, #6623, #8345, #7521, #1991, #7415, #6669, #1941, #3436, #5146, #6720, #1167, #4319, #9756, #1218, #2710, #9853, #3639, #8297, #5044, #2040, #2661, #8983, #9080, #1264, #493, #343, #7469, #4473, #1895, #3543, #9808, #5905, #6774, #6008, #2091, #8189, #1121, #4267, #4369, #3493, #5853, #9030, #9959, #5091, #445, #8239, #3586, #2811, #5957, #9137, #4422, #7572, #2862, #9186, #5240, #6940, #10110, #7787, #8609, #5352, #4730, #655, #3071, #548, #757, #1378, #9231, #7829, #6884, #3804, #9446, #10004, #4529, #3748, #7686, #2352, #4580, #8504, #2965, #5502, #10207, #8451, #6113, #2250, #3022, #602, #1532, #9341, #10053, #9291, #4681, #6165, #5294, #5397, #1430, #8661, #6997, #1582, #3696, #8555, #7737, #2912, #2303, #6830, #2204, #5448, #4629, #1481 ),
 ( #709, #3856, #10157, #6214, #6056, #9390, #3904, #7048, #3120, #6261, #2147, #4931, #9691, #9647, #4156, #6513, #2600, #856, #1008, #4107, #3951, #2449, #3380, #908, #9495, #122, #5743, #7305, #3178, #5549, #1733, #24, #2553, #1828, #4008, #5697, #4882, #6415, #1630, #4056, #6364, #7876, #9594, #957, #5595, #8758, #803, #5650, #7155, #73, #7926, #8708, #174, #8078, #8912, #8865, #227, #7097, #6314, #3227, #2400, #7251, #4777, #1685, #9542, #7203, #4828, #3274, #7981, #2501, #8819, #8026, #3332, #6469, #1778, #9842, #6562, #3573, #9174, #8129, #382, #6707, #2026, #8972, #5842, #2850, #5995, #5077, #1111, #1929, #5184, #7557, #3622, #3424, #9945, #4983, #9020, #7356, #1884, #4255, #8333, #4204, #1154, #7404, #5890, #9069, #8227, #4305, #7456, #9891, #3534, #1251, #6659, #2745, #1977, #5135, #2794, #9797, #1063, #8282, #7507, #279, #4408, #5797, #9742, #480, #328, #1204, #6759, #2649, #5032 ),
 ( #5944, #3477, #9124, #8177, #6610, #2701, #4355, #432, #5434, #3792, #4616, #5384, #2899, #8544, #4667, #10097, #5338, #8493, #1520, #7818, #6922, #8439, #9219, #6982, #5228, #5276, #8593, #698, #3845, #9328, #745, #1363, #3684, #4516, #3058, #589, #10145, #3008, #2238, #1305, #2080, #6202, #6819, #1467, #3892, #9377, #7771, #2134, #1419, #4457, #10040, #6251, #8382, #7036, #2952, #2291, #10196, #7614, #535, #7673, #9993, #6152, #3111, #3734, #6043, #6870, #6096, #9277, #2191, #4569, #7723, #643, #1619, #2388, #4767, #2485, #9580, #61, #3998, #3317, #7913, #840, #5639, #3217, #7143, #7294, #5686, #6404, #1766, #8066, #1669, #160, #7192, #2540, #5538, #791, #9636, #6353, #7968, #217, #898, #994, #8806, #4046, #9532, #8746, #6457, #2437, #109, #4143, #8697, #3368, #8015, #4818, #4093, #5583, #947, #7242, #3262, #7085, #1724, #9428, #8856, #4870, #4921, #2339, #7, #5491, #8649, #1572, #4718 ),
 ( #7864, #6302, #3941, #3164, #9485, #8901, #7444, #6550, #4289, #8163, #2634, #7344, #1192, #371, #3520, #9682, #4342, #9733, #8121, #6694, #1869, #5065, #4396, #8213, #5174, #5879, #1143, #1098, #5830, #7495, #3458, #6648, #8324, #5782, #1242, #5115, #9006, #421, #5017, #8269, #3564, #8957, #4195, #9786, #7545, #9879, #9833, #9057, #2733, #267, #1965, #9109, #2783, #2687, #1917, #5931, #2017, #471, #4239, #3414, #6502, #2589, #7390, #1815, #5734, #317, #4972, #6600, #1051, #4448, #8532, #1407, #4560, #6743, #1458, #9936, #6806, #6971, #2230, #5376, #632, #10133, #2889, #5219, #6031, #4608, #2123, #7759, #7711, #3780, #2839, #3612, #684, #8371, #6912, #2278, #3833, #10082, #524, #10031, #5983, #1351, #7810, #9162, #3049, #4506, #6191, #9317, #2069, #1292, #3672, #7599, #2998, #9366, #9983, #5425, #8582, #9211, #5263, #1505, #8423, #4658, #7660, #578, #3723, #6859, #6141, #2942, #6085, #9262, #2184 ),
 ( #5327, #8483, #3208, #9571, #6342, #4081, #7134, #50, #9522, #1561, #8794, #2428, #8640, #4707, #1714, #829, #5479, #5574, #8687, #5679, #7184, #8848, #3883, #8737, #7904, #3100, #2474, #4909, #3930, #5628, #4807, #1657, #7856, #3985, #9476, #735, #7958, #4038, #1609, #4760, #7026, #888, #3772, #3150, #780, #7074, #3253, #8006, #2530, #4859, #7231, #9627, #1758, #6290, #151, #99, #10184, #5528, #6447, #6393, #2330, #936, #6240, #3306, #9418, #2377, #2042, #1220, #8395, #2813, #9673, #6777, #2148, #985, #3588, #9960, #5241, #1805, #8946, #6057, #9232, #8298, #4185, #5148, #1320, #550, #6831, #6495, #2913, #8055, #1859, #210, #4960, #7335, #4474, #7286, #4370, #259, #9138, #5198, #7523, #446, #6721, #2863, #9906, #7630, #5959, #8347, #1265, #4424, #6009, #2625, #4134, #7573, #495, #3360, #3697, #8893, #2582, #10005, #3406, #3640, #5725, #8112, #1041, #6542, #9721, #5771, #9187, #2092, #7738 ) ),
 .UNSPECIFIED., .T., .F., .F. ) 
 B_SPLINE_SURFACE_WITH_KNOTS ( ( 4, 3, 4 ),
 ( 3, 2, 2, 2, 2, 2, 2, 2, 2, 2, 2, 2, 2, 2, 2, 2, 2, 2, 2, 2, 2, 2, 2, 2, 2, 2, 2, 2, 2, 2, 2, 2, 2, 2, 2, 2, 2, 2, 2, 2, 2, 2, 2, 2, 2, 2, 2, 2, 2, 2, 2, 2, 2, 2, 2, 2, 2, 2, 2, 2, 2, 2, 2, 2, 2, 3 ),
 ( 0.000000000000000000, 0.5000000000000000000, 1.000000000000000000 ),
 ( 0.000000000000000000, 0.01428571428571428527, 0.02857142857142857054, 0.04285714285714285754, 0.05714285714285714107, 0.07142857142857142461, 0.08571428571428571508, 0.1000000000000000056, 0.1142857142857142821, 0.1285714285714285587, 0.1428571428571428492, 0.1571428571428571397, 0.1714285714285714302, 0.1857142857142857206, 0.2000000000000000111, 0.2142857142857142738, 0.2285714285714285643, 0.2428571428571428548, 0.2571428571428571175, 0.2714285714285714080, 0.2857142857142856984, 0.2999999999999999889, 0.3142857142857142794, 0.3285714285714285698, 0.3428571428571428603, 0.3571428571428571508, 0.3714285714285714413, 0.3857142857142857317, 0.4000000000000000222, 0.4142857142857143127, 0.4285714285714285476, 0.4428571428571428381, 0.4571428571428571286, 0.4714285714285714191, 0.4857142857142857095, 0.5000000000000000000, 0.5142857142857142350, 0.5285714285714285809, 0.5428571428571428159, 0.5571428571428571619, 0.5714285714285713969, 0.5857142857142857428, 0.5999999999999999778, 0.6142857142857143238, 0.6285714285714285587, 0.6428571428571429047, 0.6571428571428571397, 0.6714285714285713746, 0.6857142857142857206, 0.6999999999999999556, 0.7142857142857143016, 0.7285714285714285365, 0.7428571428571428825, 0.7571428571428571175, 0.7714285714285714635, 0.7857142857142856984, 0.8000000000000000444, 0.8142857142857142794, 0.8285714285714286254, 0.8428571428571428603, 0.8571428571428570953, 0.8714285714285714413, 0.8857142857142856762, 0.9000000000000000222, 0.9142857142857142572, 0.9285714285714286031 ),
 .UNSPECIFIED. ) 
 GEOMETRIC_REPRESENTATION_ITEM ( )  RATIONAL_B_SPLINE_SURFACE ( (
 ( 1.000000000000000000, 0.9510565162951535312, 1.000000000000000000, 0.9510565162951535312, 1.000000000000000000, 0.9510565162951535312, 1.000000000000000000, 0.9510565162951535312, 1.000000000000000000, 0.9510565162951535312, 1.000000000000000000, 0.9510565162951535312, 1.000000000000000000, 0.9510565162951535312, 1.000000000000000000, 0.9510565162951535312, 1.000000000000000000, 0.9510565162951535312, 1.000000000000000000, 0.9510565162951535312, 1.000000000000000000, 0.9510565162951535312, 1.000000000000000000, 0.9510565162951535312, 1.000000000000000000, 0.9510565162951535312, 1.000000000000000000, 0.9510565162951535312, 1.000000000000000000, 0.9510565162951535312, 1.000000000000000000, 0.9510565162951535312, 1.000000000000000000, 0.9510565162951535312, 1.000000000000000000, 0.9510565162951535312, 1.000000000000000000, 0.9510565162951535312, 1.000000000000000000, 0.9510565162951535312, 1.000000000000000000, 0.9510565162951535312, 1.000000000000000000, 0.9510565162951535312, 1.000000000000000000, 0.9510565162951535312, 1.000000000000000000, 0.9510565162951535312, 1.000000000000000000, 0.9510565162951535312, 1.000000000000000000, 0.9510565162951535312, 1.000000000000000000, 0.9510565162951535312, 1.000000000000000000, 0.9510565162951535312, 1.000000000000000000, 0.9510565162951535312, 1.000000000000000000, 0.9510565162951535312, 1.000000000000000000, 0.9510565162951535312, 1.000000000000000000, 0.9510565162951535312, 1.000000000000000000, 0.9510565162951535312, 1.000000000000000000, 0.9510565162951535312, 1.000000000000000000, 0.9510565162951535312, 1.000000000000000000, 0.9510565162951535312, 1.000000000000000000, 0.9510565162951535312, 1.000000000000000000, 0.9510565162951535312, 1.000000000000000000, 0.9510565162951535312, 1.000000000000000000, 0.9510565162951535312, 1.000000000000000000, 0.9510565162951535312, 1.000000000000000000, 0.9510565162951535312, 1.000000000000000000, 0.9510565162951535312, 1.000000000000000000, 0.9510565162951535312, 1.000000000000000000, 0.9510565162951535312, 1.000000000000000000, 0.9510565162951535312, 1.000000000000000000, 0.9510565162951535312, 1.000000000000000000, 0.9510565162951535312, 1.000000000000000000, 0.9510565162951535312, 1.000000000000000000, 0.9510565162951535312, 1.000000000000000000, 0.9510565162951535312, 1.000000000000000000, 0.9510565162951535312, 1.000000000000000000, 0.9510565162951535312, 1.000000000000000000, 0.9510565162951535312, 1.000000000000000000, 0.9510565162951535312, 1.000000000000000000, 0.9510565162951535312, 1.000000000000000000, 0.9510565162951535312, 1.000000000000000000, 0.9510565162951535312, 1.000000000000000000, 0.9510565162951535312, 1.000000000000000000, 0.9510565162951535312, 1.000000000000000000, 0.9510565162951535312, 1.000000000000000000, 0.9510565162951535312, 1.000000000000000000, 0.9510565162951535312, 1.000000000000000000, 0.9510565162951535312, 1.000000000000000000, 0.9510565162951535312, 1.000000000000000000),
 ( 0.3333333333333333703, 0.3170188387650512141, 0.3333333333333333703, 0.3170188387650512141, 0.3333333333333333703, 0.3170188387650512141, 0.3333333333333333703, 0.3170188387650512141, 0.3333333333333333703, 0.3170188387650512141, 0.3333333333333333703, 0.3170188387650512141, 0.3333333333333333703, 0.3170188387650512141, 0.3333333333333333703, 0.3170188387650512141, 0.3333333333333333703, 0.3170188387650512141, 0.3333333333333333703, 0.3170188387650512141, 0.3333333333333333703, 0.3170188387650512141, 0.3333333333333333703, 0.3170188387650512141, 0.3333333333333333703, 0.3170188387650512141, 0.3333333333333333703, 0.3170188387650512141, 0.3333333333333333703, 0.3170188387650512141, 0.3333333333333333703, 0.3170188387650512141, 0.3333333333333333703, 0.3170188387650512141, 0.3333333333333333703, 0.3170188387650512141, 0.3333333333333333703, 0.3170188387650512141, 0.3333333333333333703, 0.3170188387650512141, 0.3333333333333333703, 0.3170188387650512141, 0.3333333333333333703, 0.3170188387650512141, 0.3333333333333333703, 0.3170188387650512141, 0.3333333333333333703, 0.3170188387650512141, 0.3333333333333333703, 0.3170188387650512141, 0.3333333333333333703, 0.3170188387650512141, 0.3333333333333333703, 0.3170188387650512141, 0.3333333333333333703, 0.3170188387650512141, 0.3333333333333333703, 0.3170188387650512141, 0.3333333333333333703, 0.3170188387650512141, 0.3333333333333333703, 0.3170188387650512141, 0.3333333333333333703, 0.3170188387650512141, 0.3333333333333333703, 0.3170188387650512141, 0.3333333333333333703, 0.3170188387650512141, 0.3333333333333333703, 0.3170188387650512141, 0.3333333333333333703, 0.3170188387650512141, 0.3333333333333333703, 0.3170188387650512141, 0.3333333333333333703, 0.3170188387650512141, 0.3333333333333333703, 0.3170188387650512141, 0.3333333333333333703, 0.3170188387650512141, 0.3333333333333333703, 0.3170188387650512141, 0.3333333333333333703, 0.3170188387650512141, 0.3333333333333333703, 0.3170188387650512141, 0.3333333333333333703, 0.3170188387650512141, 0.3333333333333333703, 0.3170188387650512141, 0.3333333333333333703, 0.3170188387650512141, 0.3333333333333333703, 0.3170188387650512141, 0.3333333333333333703, 0.3170188387650512141, 0.3333333333333333703, 0.3170188387650512141, 0.3333333333333333703, 0.3170188387650512141, 0.3333333333333333703, 0.3170188387650512141, 0.3333333333333333703, 0.3170188387650512141, 0.3333333333333333703, 0.3170188387650512141, 0.3333333333333333703, 0.3170188387650512141, 0.3333333333333333703, 0.3170188387650512141, 0.3333333333333333703, 0.3170188387650512141, 0.3333333333333333703, 0.3170188387650512141, 0.3333333333333333703, 0.3170188387650512141, 0.3333333333333333703, 0.3170188387650512141, 0.3333333333333333703, 0.3170188387650512141, 0.3333333333333333703, 0.3170188387650512141, 0.3333333333333333703, 0.3170188387650512141, 0.3333333333333333703, 0.3170188387650512141, 0.3333333333333333703, 0.3170188387650512141, 0.3333333333333333703, 0.3170188387650512141, 0.3333333333333333703),
 ( 0.3333333333333333703, 0.3170188387650512141, 0.3333333333333333703, 0.3170188387650512141, 0.3333333333333333703, 0.3170188387650512141, 0.3333333333333333703, 0.3170188387650512141, 0.3333333333333333703, 0.3170188387650512141, 0.3333333333333333703, 0.3170188387650512141, 0.3333333333333333703, 0.3170188387650512141, 0.3333333333333333703, 0.3170188387650512141, 0.3333333333333333703, 0.3170188387650512141, 0.3333333333333333703, 0.3170188387650512141, 0.3333333333333333703, 0.3170188387650512141, 0.3333333333333333703, 0.3170188387650512141, 0.3333333333333333703, 0.3170188387650512141, 0.3333333333333333703, 0.3170188387650512141, 0.3333333333333333703, 0.3170188387650512141, 0.3333333333333333703, 0.3170188387650512141, 0.3333333333333333703, 0.3170188387650512141, 0.3333333333333333703, 0.3170188387650512141, 0.3333333333333333703, 0.3170188387650512141, 0.3333333333333333703, 0.3170188387650512141, 0.3333333333333333703, 0.3170188387650512141, 0.3333333333333333703, 0.3170188387650512141, 0.3333333333333333703, 0.3170188387650512141, 0.3333333333333333703, 0.3170188387650512141, 0.3333333333333333703, 0.3170188387650512141, 0.3333333333333333703, 0.3170188387650512141, 0.3333333333333333703, 0.3170188387650512141, 0.3333333333333333703, 0.3170188387650512141, 0.3333333333333333703, 0.3170188387650512141, 0.3333333333333333703, 0.3170188387650512141, 0.3333333333333333703, 0.3170188387650512141, 0.3333333333333333703, 0.3170188387650512141, 0.3333333333333333703, 0.3170188387650512141, 0.3333333333333333703, 0.3170188387650512141, 0.3333333333333333703, 0.3170188387650512141, 0.3333333333333333703, 0.3170188387650512141, 0.3333333333333333703, 0.3170188387650512141, 0.3333333333333333703, 0.3170188387650512141, 0.3333333333333333703, 0.3170188387650512141, 0.3333333333333333703, 0.3170188387650512141, 0.3333333333333333703, 0.3170188387650512141, 0.3333333333333333703, 0.3170188387650512141, 0.3333333333333333703, 0.3170188387650512141, 0.3333333333333333703, 0.3170188387650512141, 0.3333333333333333703, 0.3170188387650512141, 0.3333333333333333703, 0.3170188387650512141, 0.3333333333333333703, 0.3170188387650512141, 0.3333333333333333703, 0.3170188387650512141, 0.3333333333333333703, 0.3170188387650512141, 0.3333333333333333703, 0.3170188387650512141, 0.3333333333333333703, 0.3170188387650512141, 0.3333333333333333703, 0.3170188387650512141, 0.3333333333333333703, 0.3170188387650512141, 0.3333333333333333703, 0.3170188387650512141, 0.3333333333333333703, 0.3170188387650512141, 0.3333333333333333703, 0.3170188387650512141, 0.3333333333333333703, 0.3170188387650512141, 0.3333333333333333703, 0.3170188387650512141, 0.3333333333333333703, 0.3170188387650512141, 0.3333333333333333703, 0.3170188387650512141, 0.3333333333333333703, 0.3170188387650512141, 0.3333333333333333703, 0.3170188387650512141, 0.3333333333333333703, 0.3170188387650512141, 0.3333333333333333703, 0.3170188387650512141, 0.3333333333333333703, 0.3170188387650512141, 0.3333333333333333703),
 ( 1.000000000000000000, 0.9510565162951535312, 1.000000000000000000, 0.9510565162951535312, 1.000000000000000000, 0.9510565162951535312, 1.000000000000000000, 0.9510565162951535312, 1.000000000000000000, 0.9510565162951535312, 1.000000000000000000, 0.9510565162951535312, 1.000000000000000000, 0.9510565162951535312, 1.000000000000000000, 0.9510565162951535312, 1.000000000000000000, 0.9510565162951535312, 1.000000000000000000, 0.9510565162951535312, 1.000000000000000000, 0.9510565162951535312, 1.000000000000000000, 0.9510565162951535312, 1.000000000000000000, 0.9510565162951535312, 1.000000000000000000, 0.9510565162951535312, 1.000000000000000000, 0.9510565162951535312, 1.000000000000000000, 0.9510565162951535312, 1.000000000000000000, 0.9510565162951535312, 1.000000000000000000, 0.9510565162951535312, 1.000000000000000000, 0.9510565162951535312, 1.000000000000000000, 0.9510565162951535312, 1.000000000000000000, 0.9510565162951535312, 1.000000000000000000, 0.9510565162951535312, 1.000000000000000000, 0.9510565162951535312, 1.000000000000000000, 0.9510565162951535312, 1.000000000000000000, 0.9510565162951535312, 1.000000000000000000, 0.9510565162951535312, 1.000000000000000000, 0.9510565162951535312, 1.000000000000000000, 0.9510565162951535312, 1.000000000000000000, 0.9510565162951535312, 1.000000000000000000, 0.9510565162951535312, 1.000000000000000000, 0.9510565162951535312, 1.000000000000000000, 0.9510565162951535312, 1.000000000000000000, 0.9510565162951535312, 1.000000000000000000, 0.9510565162951535312, 1.000000000000000000, 0.9510565162951535312, 1.000000000000000000, 0.9510565162951535312, 1.000000000000000000, 0.9510565162951535312, 1.000000000000000000, 0.9510565162951535312, 1.000000000000000000, 0.9510565162951535312, 1.000000000000000000, 0.9510565162951535312, 1.000000000000000000, 0.9510565162951535312, 1.000000000000000000, 0.9510565162951535312, 1.000000000000000000, 0.9510565162951535312, 1.000000000000000000, 0.9510565162951535312, 1.000000000000000000, 0.9510565162951535312, 1.000000000000000000, 0.9510565162951535312, 1.000000000000000000, 0.9510565162951535312, 1.000000000000000000, 0.9510565162951535312, 1.000000000000000000, 0.9510565162951535312, 1.000000000000000000, 0.9510565162951535312, 1.000000000000000000, 0.9510565162951535312, 1.000000000000000000, 0.9510565162951535312, 1.000000000000000000, 0.9510565162951535312, 1.000000000000000000, 0.9510565162951535312, 1.000000000000000000, 0.9510565162951535312, 1.000000000000000000, 0.9510565162951535312, 1.000000000000000000, 0.9510565162951535312, 1.000000000000000000, 0.9510565162951535312, 1.000000000000000000, 0.9510565162951535312, 1.000000000000000000, 0.9510565162951535312, 1.000000000000000000, 0.9510565162951535312, 1.000000000000000000, 0.9510565162951535312, 1.000000000000000000, 0.9510565162951535312, 1.000000000000000000, 0.9510565162951535312, 1.000000000000000000, 0.9510565162951535312, 1.000000000000000000),
 ( 0.3333333333333333703, 0.3170188387650512141, 0.3333333333333333703, 0.3170188387650512141, 0.3333333333333333703, 0.3170188387650512141, 0.3333333333333333703, 0.3170188387650512141, 0.3333333333333333703, 0.3170188387650512141, 0.3333333333333333703, 0.3170188387650512141, 0.3333333333333333703, 0.3170188387650512141, 0.3333333333333333703, 0.3170188387650512141, 0.3333333333333333703, 0.3170188387650512141, 0.3333333333333333703, 0.3170188387650512141, 0.3333333333333333703, 0.3170188387650512141, 0.3333333333333333703, 0.3170188387650512141, 0.3333333333333333703, 0.3170188387650512141, 0.3333333333333333703, 0.3170188387650512141, 0.3333333333333333703, 0.3170188387650512141, 0.3333333333333333703, 0.3170188387650512141, 0.3333333333333333703, 0.3170188387650512141, 0.3333333333333333703, 0.3170188387650512141, 0.3333333333333333703, 0.3170188387650512141, 0.3333333333333333703, 0.3170188387650512141, 0.3333333333333333703, 0.3170188387650512141, 0.3333333333333333703, 0.3170188387650512141, 0.3333333333333333703, 0.3170188387650512141, 0.3333333333333333703, 0.3170188387650512141, 0.3333333333333333703, 0.3170188387650512141, 0.3333333333333333703, 0.3170188387650512141, 0.3333333333333333703, 0.3170188387650512141, 0.3333333333333333703, 0.3170188387650512141, 0.3333333333333333703, 0.3170188387650512141, 0.3333333333333333703, 0.3170188387650512141, 0.3333333333333333703, 0.3170188387650512141, 0.3333333333333333703, 0.3170188387650512141, 0.3333333333333333703, 0.3170188387650512141, 0.3333333333333333703, 0.3170188387650512141, 0.3333333333333333703, 0.3170188387650512141, 0.3333333333333333703, 0.3170188387650512141, 0.3333333333333333703, 0.3170188387650512141, 0.3333333333333333703, 0.3170188387650512141, 0.3333333333333333703, 0.3170188387650512141, 0.3333333333333333703, 0.3170188387650512141, 0.3333333333333333703, 0.3170188387650512141, 0.3333333333333333703, 0.3170188387650512141, 0.3333333333333333703, 0.3170188387650512141, 0.3333333333333333703, 0.3170188387650512141, 0.3333333333333333703, 0.3170188387650512141, 0.3333333333333333703, 0.3170188387650512141, 0.3333333333333333703, 0.3170188387650512141, 0.3333333333333333703, 0.3170188387650512141, 0.3333333333333333703, 0.3170188387650512141, 0.3333333333333333703, 0.3170188387650512141, 0.3333333333333333703, 0.3170188387650512141, 0.3333333333333333703, 0.3170188387650512141, 0.3333333333333333703, 0.3170188387650512141, 0.3333333333333333703, 0.3170188387650512141, 0.3333333333333333703, 0.3170188387650512141, 0.3333333333333333703, 0.3170188387650512141, 0.3333333333333333703, 0.3170188387650512141, 0.3333333333333333703, 0.3170188387650512141, 0.3333333333333333703, 0.3170188387650512141, 0.3333333333333333703, 0.3170188387650512141, 0.3333333333333333703, 0.3170188387650512141, 0.3333333333333333703, 0.3170188387650512141, 0.3333333333333333703, 0.3170188387650512141, 0.3333333333333333703, 0.3170188387650512141, 0.3333333333333333703, 0.3170188387650512141, 0.3333333333333333703),
 ( 0.3333333333333333703, 0.3170188387650512141, 0.3333333333333333703, 0.3170188387650512141, 0.3333333333333333703, 0.3170188387650512141, 0.3333333333333333703, 0.3170188387650512141, 0.3333333333333333703, 0.3170188387650512141, 0.3333333333333333703, 0.3170188387650512141, 0.3333333333333333703, 0.3170188387650512141, 0.3333333333333333703, 0.3170188387650512141, 0.3333333333333333703, 0.3170188387650512141, 0.3333333333333333703, 0.3170188387650512141, 0.3333333333333333703, 0.3170188387650512141, 0.3333333333333333703, 0.3170188387650512141, 0.3333333333333333703, 0.3170188387650512141, 0.3333333333333333703, 0.3170188387650512141, 0.3333333333333333703, 0.3170188387650512141, 0.3333333333333333703, 0.3170188387650512141, 0.3333333333333333703, 0.3170188387650512141, 0.3333333333333333703, 0.3170188387650512141, 0.3333333333333333703, 0.3170188387650512141, 0.3333333333333333703, 0.3170188387650512141, 0.3333333333333333703, 0.3170188387650512141, 0.3333333333333333703, 0.3170188387650512141, 0.3333333333333333703, 0.3170188387650512141, 0.3333333333333333703, 0.3170188387650512141, 0.3333333333333333703, 0.3170188387650512141, 0.3333333333333333703, 0.3170188387650512141, 0.3333333333333333703, 0.3170188387650512141, 0.3333333333333333703, 0.3170188387650512141, 0.3333333333333333703, 0.3170188387650512141, 0.3333333333333333703, 0.3170188387650512141, 0.3333333333333333703, 0.3170188387650512141, 0.3333333333333333703, 0.3170188387650512141, 0.3333333333333333703, 0.3170188387650512141, 0.3333333333333333703, 0.3170188387650512141, 0.3333333333333333703, 0.3170188387650512141, 0.3333333333333333703, 0.3170188387650512141, 0.3333333333333333703, 0.3170188387650512141, 0.3333333333333333703, 0.3170188387650512141, 0.3333333333333333703, 0.3170188387650512141, 0.3333333333333333703, 0.3170188387650512141, 0.3333333333333333703, 0.3170188387650512141, 0.3333333333333333703, 0.3170188387650512141, 0.3333333333333333703, 0.3170188387650512141, 0.3333333333333333703, 0.3170188387650512141, 0.3333333333333333703, 0.3170188387650512141, 0.3333333333333333703, 0.3170188387650512141, 0.3333333333333333703, 0.3170188387650512141, 0.3333333333333333703, 0.3170188387650512141, 0.3333333333333333703, 0.3170188387650512141, 0.3333333333333333703, 0.3170188387650512141, 0.3333333333333333703, 0.3170188387650512141, 0.3333333333333333703, 0.3170188387650512141, 0.3333333333333333703, 0.3170188387650512141, 0.3333333333333333703, 0.3170188387650512141, 0.3333333333333333703, 0.3170188387650512141, 0.3333333333333333703, 0.3170188387650512141, 0.3333333333333333703, 0.3170188387650512141, 0.3333333333333333703, 0.3170188387650512141, 0.3333333333333333703, 0.3170188387650512141, 0.3333333333333333703, 0.3170188387650512141, 0.3333333333333333703, 0.3170188387650512141, 0.3333333333333333703, 0.3170188387650512141, 0.3333333333333333703, 0.3170188387650512141, 0.3333333333333333703, 0.3170188387650512141, 0.3333333333333333703, 0.3170188387650512141, 0.3333333333333333703),
 ( 1.000000000000000000, 0.9510565162951535312, 1.000000000000000000, 0.9510565162951535312, 1.000000000000000000, 0.9510565162951535312, 1.000000000000000000, 0.9510565162951535312, 1.000000000000000000, 0.9510565162951535312, 1.000000000000000000, 0.9510565162951535312, 1.000000000000000000, 0.9510565162951535312, 1.000000000000000000, 0.9510565162951535312, 1.000000000000000000, 0.9510565162951535312, 1.000000000000000000, 0.9510565162951535312, 1.000000000000000000, 0.9510565162951535312, 1.000000000000000000, 0.9510565162951535312, 1.000000000000000000, 0.9510565162951535312, 1.000000000000000000, 0.9510565162951535312, 1.000000000000000000, 0.9510565162951535312, 1.000000000000000000, 0.9510565162951535312, 1.000000000000000000, 0.9510565162951535312, 1.000000000000000000, 0.9510565162951535312, 1.000000000000000000, 0.9510565162951535312, 1.000000000000000000, 0.9510565162951535312, 1.000000000000000000, 0.9510565162951535312, 1.000000000000000000, 0.9510565162951535312, 1.000000000000000000, 0.9510565162951535312, 1.000000000000000000, 0.9510565162951535312, 1.000000000000000000, 0.9510565162951535312, 1.000000000000000000, 0.9510565162951535312, 1.000000000000000000, 0.9510565162951535312, 1.000000000000000000, 0.9510565162951535312, 1.000000000000000000, 0.9510565162951535312, 1.000000000000000000, 0.9510565162951535312, 1.000000000000000000, 0.9510565162951535312, 1.000000000000000000, 0.9510565162951535312, 1.000000000000000000, 0.9510565162951535312, 1.000000000000000000, 0.9510565162951535312, 1.000000000000000000, 0.9510565162951535312, 1.000000000000000000, 0.9510565162951535312, 1.000000000000000000, 0.9510565162951535312, 1.000000000000000000, 0.9510565162951535312, 1.000000000000000000, 0.9510565162951535312, 1.000000000000000000, 0.9510565162951535312, 1.000000000000000000, 0.9510565162951535312, 1.000000000000000000, 0.9510565162951535312, 1.000000000000000000, 0.9510565162951535312, 1.000000000000000000, 0.9510565162951535312, 1.000000000000000000, 0.9510565162951535312, 1.000000000000000000, 0.9510565162951535312, 1.000000000000000000, 0.9510565162951535312, 1.000000000000000000, 0.9510565162951535312, 1.000000000000000000, 0.9510565162951535312, 1.000000000000000000, 0.9510565162951535312, 1.000000000000000000, 0.9510565162951535312, 1.000000000000000000, 0.9510565162951535312, 1.000000000000000000, 0.9510565162951535312, 1.000000000000000000, 0.9510565162951535312, 1.000000000000000000, 0.9510565162951535312, 1.000000000000000000, 0.9510565162951535312, 1.000000000000000000, 0.9510565162951535312, 1.000000000000000000, 0.9510565162951535312, 1.000000000000000000, 0.9510565162951535312, 1.000000000000000000, 0.9510565162951535312, 1.000000000000000000, 0.9510565162951535312, 1.000000000000000000, 0.9510565162951535312, 1.000000000000000000, 0.9510565162951535312, 1.000000000000000000, 0.9510565162951535312, 1.000000000000000000, 0.9510565162951535312, 1.000000000000000000) ) ) 
 REPRESENTATION_ITEM ( '' )  SURFACE ( )  );
#1123=PRODUCT_DEFINITION_CONTEXT ( 'detailed design', #4679, 'design' ) ;
#1127=CARTESIAN_POINT ( 'NONE',  ( 6.717514421272239744, -6.717514421272154479, 16.50000000000001421 ) ) ;
#1128=CARTESIAN_POINT ( 'NONE',  ( 1.689666864740335894, -10.36326688006720786, 5.798862081921429379 ) ) ;
#1135=CARTESIAN_POINT ( 'NONE',  ( 7.424621202458790314, -7.424621202458697944, 4.500000000000003553 ) ) ;
#1139=VERTEX_POINT ( 'NONE', #7937 ) ;
#1142=CARTESIAN_POINT ( 'NONE',  ( -7.390897758835869524, 7.458344646081637386, 14.00113791807859620 ) ) ;
#1143=CARTESIAN_POINT ( 'NONE',  ( 9.377220287599001836, 4.724406229267492208, 2.901137918078569466 ) ) ;
#1147=CARTESIAN_POINT ( 'NONE',  ( -7.424621202458789426, 7.424621202458724589, 12.00000000000001066 ) ) ;
#1153=CARTESIAN_POINT ( 'NONE',  ( 9.873755945037075321, 1.513077731353043243, 3.051137918078546285 ) ) ;
#1154=CARTESIAN_POINT ( 'NONE',  ( -1.486127417882243895, 9.383039235653816590, 15.29999999999997939 ) ) ;
#1166=CARTESIAN_POINT ( 'NONE',  ( 7.027753727702739539, 7.098671581784288698, 16.74886208192143755 ) ) ;
#1167=CARTESIAN_POINT ( 'NONE',  ( -1.513077731352923339, -9.873755945037078874, 5.948862081921430622 ) ) ;
#1183=CARTESIAN_POINT ( 'NONE',  ( 9.355568503977840678, 4.766900247265305701, 18.90000000000002700 ) ) ;
#1189=CARTESIAN_POINT ( 'NONE',  ( 8.442910196168311288, 4.355403765523574222, 4.898862081921403266 ) ) ;
#1191=CARTESIAN_POINT ( 'NONE',  ( 9.355568503977840678, 4.766900247265305701, 3.899999999999959055 ) ) ;
#1192=CARTESIAN_POINT ( 'NONE',  ( 1.595456901104624459, -10.37818827243064668, 0.8011379180785925813 ) ) ;
#1196=CARTESIAN_POINT ( 'NONE',  ( 1.642561882922480621, -10.37072757624891750, 7.800000000000029132 ) ) ;
#1203=CARTESIAN_POINT ( 'NONE',  ( -8.877401133907129704, 4.579542530753042406, 7.851137918078569200 ) ) ;
#1204=CARTESIAN_POINT ( 'NONE',  ( 9.865911304835474738, 1.562606840307950051, 19.04999999999997939 ) ) ;
#1217=CARTESIAN_POINT ( 'NONE',  ( -1.533232399700100057, 9.375578539472094519, 19.29886208192143471 ) ) ;
#1218=CARTESIAN_POINT ( 'NONE',  ( -8.442910196168309511, -4.355403765523546689, 6.398862081921404155 ) ) ;
#1220=CARTESIAN_POINT ( 'NONE',  ( 10.90442828429183919, 1.727091770866679532, 10.05000000000002736 ) ) ;
#1233=CARTESIAN_POINT ( 'NONE',  ( -1.727091770866549414, -10.90442828429184630, 16.94999999999998863 ) ) ;
#1239=CARTESIAN_POINT ( 'NONE',  ( -10.37818827243067688, 1.595456901104524761, 18.69886208192145816 ) ) ;
#1241=CARTESIAN_POINT ( 'NONE',  ( 10.37072757624895836, -1.642561882922355609, 4.199999999999981526 ) ) ;
#1242=CARTESIAN_POINT ( 'NONE',  ( -4.809394265263009061, -9.333916720356723928, 4.101137918078561206 ) ) ;
#1245=CARTESIAN_POINT ( 'NONE',  ( -7.806708723663830618, -7.806708723663901672, 5.250000000000008882 ) ) ;
#1250=CARTESIAN_POINT ( 'NONE',  ( -9.873755945037078874, -1.513077731353019706, 13.55113791807856316 ) ) ;
#1251=CARTESIAN_POINT ( 'NONE',  ( 4.534861676072320158, -8.900167166472098046, 16.64999999999999858 ) ) ;
#1262=CARTESIAN_POINT ( 'NONE',  ( -1.727091770866549414, -10.90442828429184630, 1.949999999999996181 ) ) ;
#1263=CARTESIAN_POINT ( 'NONE',  ( 8.900167166472154889, -4.534861676072210024, 10.35000000000002274 ) ) ;
#1264=CARTESIAN_POINT ( 'NONE',  ( 8.442910196168311288, 4.355403765523576887, 7.898862081921404155 ) ) ;
#1265=CARTESIAN_POINT ( 'NONE',  ( 10.37072757624895836, -1.642561882922356498, 16.19999999999999218 ) ) ;
#1275=CARTESIAN_POINT ( 'NONE',  ( -9.355568503977838901, -4.766900247265279944, 17.39999999999997016 ) ) ;
#1277=AXIS2_PLACEMENT_3D ( 'NONE', #1556, #518, #6800 ) ;
#1279=( GEOMETRIC_REPRESENTATION_CONTEXT ( 3 ) GLOBAL_UNCERTAINTY_ASSIGNED_CONTEXT ( ( #2663 ) ) GLOBAL_UNIT_ASSIGNED_CONTEXT ( ( #102, #6345, #938 ) ) REPRESENTATION_CONTEXT ( 'NONE', 'WORKASPACE' ) );
#1281=CARTESIAN_POINT ( 'NONE',  ( -9.355568503977838901, -4.766900247265280832, 14.39999999999996838 ) ) ;
#1287=CARTESIAN_POINT ( 'NONE',  ( 4.766900247265192903, 9.355568503977902850, 18.60000000000000497 ) ) ;
#1289=CARTESIAN_POINT ( 'NONE',  ( -10.37818827243067688, 1.595456901104524761, 15.69886208192145816 ) ) ;
#1291=CARTESIAN_POINT ( 'NONE',  ( -10.37072757624895836, 1.642561882922381145, 8.700000000000041922 ) ) ;
#1292=CARTESIAN_POINT ( 'NONE',  ( 9.814260835641038128, -5.056896391392198709, 15.35113791807859229 ) ) ;
#1298=CARTESIAN_POINT ( 'NONE',  ( 1.727091770866550968, 10.90442828429187294, 9.449999999999988631 ) ) ;
#1304=CARTESIAN_POINT ( 'NONE',  ( 9.375578539472099848, -1.533232399699986370, 18.20113791807854398 ) ) ;
#1305=CARTESIAN_POINT ( 'NONE',  ( -8.877401133907129704, 4.579542530753042406, 4.851137918078532785 ) ) ;
#1318=CARTESIAN_POINT ( 'NONE',  ( -1.562606840307830591, -9.865911304835476514, 7.950000000000040146 ) ) ;
#1319=CARTESIAN_POINT ( 'NONE',  ( -8.442910196168309511, -4.355403765523544024, 3.398862081921444123 ) ) ;
#1320=CARTESIAN_POINT ( 'NONE',  ( 4.766900247265192903, 9.355568503977902850, 12.59999999999999964 ) ) ;
#1323=AXIS2_PLACEMENT_3D ( 'NONE', #6239, #7957, #5375 ) ;
#1328=CARTESIAN_POINT ( 'NONE',  ( 5.012215536711511987, -9.837026868205999364, 16.64999999999999858 ) ) ;
#1329=ORIENTED_EDGE ( 'NONE', *, *, #7762, .T. ) ;
#1335=CARTESIAN_POINT ( 'NONE',  ( 9.837026868206066865, -5.012215536711392083, 19.34999999999996945 ) ) ;
#1346=FACE_OUTER_BOUND ( 'NONE', #2854, .T. ) ;
#1348=CARTESIAN_POINT ( 'NONE',  ( 10.37818827243067510, -1.595456901104499225, 20.19886208192146526 ) ) ;
#1350=CARTESIAN_POINT ( 'NONE',  ( 1.642561882922480621, -10.37072757624892638, 1.800000000000023803 ) ) ;
#1351=CARTESIAN_POINT ( 'NONE',  ( -4.967534682030703586, 9.859792900771058299, 14.15113791807854327 ) ) ;
#1355=CARTESIAN_POINT ( 'NONE',  ( -9.333916720356675967, -4.809394265263095214, 3.398862081921444123 ) ) ;
#1358=CARTESIAN_POINT ( 'NONE',  ( 7.806708723663832394, 7.806708723663930982, 6.749999999999960920 ) ) ;
#1362=CARTESIAN_POINT ( 'NONE',  ( 4.809394265263009061, 9.333916720356739916, -0.3988620819214416247 ) ) ;
#1363=CARTESIAN_POINT ( 'NONE',  ( 4.490180821391514421, -8.922933199037139218, 3.651137918078570355 ) ) ;
#1376=CARTESIAN_POINT ( 'NONE',  ( 9.837026868206066865, -5.012215536711392083, 1.350000000000015188 ) ) ;
#1377=CARTESIAN_POINT ( 'NONE',  ( 1.562606840307832368, 9.865911304835510265, 3.450000000000006839 ) ) ;
#1378=CARTESIAN_POINT ( 'NONE',  ( 9.390499931835536884, -1.439022436064273158, 14.19886208192146171 ) ) ;
#1387=CARTESIAN_POINT ( 'NONE',  ( -1.642561882922479732, 10.37072757624895303, 12.29999999999997762 ) ) ;
#1392=CARTESIAN_POINT ( 'NONE',  ( 7.458344646081711105, -7.390897758835786036, 2.498862081921459755 ) ) ;
#1404=CARTESIAN_POINT ( 'NONE',  ( 7.027753727702739539, 7.098671581784288698, 7.748862081921418010 ) ) ;
#1406=CARTESIAN_POINT ( 'NONE',  ( -10.37072757624895836, 1.642561882922381145, 5.700000000000038369 ) ) ;
#1407=CARTESIAN_POINT ( 'NONE',  ( 4.967534682030706250, -9.859792900771036983, 9.651137918078598332 ) ) ;
#1413=CARTESIAN_POINT ( 'NONE',  ( -9.355568503977838901, -4.766900247265280832, 2.400000000000013234 ) ) ;
#1414=EDGE_CURVE ( 'NONE', #7327, #8995, #6320, .T. ) ;
#1418=CARTESIAN_POINT ( 'NONE',  ( -1.439022436064386845, 9.390499931835526226, 11.30113791807855961 ) ) ;
#1419=CARTESIAN_POINT ( 'NONE',  ( 9.375578539472099848, -1.533232399699986370, 6.201137918078538647 ) ) ;
#1428=CARTESIAN_POINT ( 'NONE',  ( -6.717514421272238856, 6.717514421272181124, 2.585396704745767526E-18 ) ) ;
#1429=CARTESIAN_POINT ( 'NONE',  ( -6.717514421272238856, 6.717514421272181124, 12.00000000000001066 ) ) ;
#1430=CARTESIAN_POINT ( 'NONE',  ( -9.858066664633883036, -1.612135949262831547, 18.54886208192142405 ) ) ;
#1437=CARTESIAN_POINT ( 'NONE',  ( 5.012215536711511987, -9.837026868205999364, 10.65000000000000924 ) ) ;
#1442=CARTESIAN_POINT ( 'NONE',  ( -10.37818827243067688, 1.595456901104523428, 12.69886208192145816 ) ) ;
#1448=CARTESIAN_POINT ( 'NONE',  ( -8.900167166472160218, 4.534861676072235781, 5.849999999999989875 ) ) ;
#1458=CARTESIAN_POINT ( 'NONE',  ( -4.809394265263009061, -9.333916720356718599, 10.10113791807856742 ) ) ;
#1463=CARTESIAN_POINT ( 'NONE',  ( -7.424621202458789426, 7.424621202458724589, 6.000000000000005329 ) ) ;
#1466=CARTESIAN_POINT ( 'NONE',  ( 7.098671581784200768, 7.027753727702831021, 11.75113791807857666 ) ) ;
#1467=CARTESIAN_POINT ( 'NONE',  ( 1.612135949262739398, 9.858066664633913234, 5.451137918078557298 ) ) ;
#1480=CARTESIAN_POINT ( 'NONE',  ( -6.717514421272238856, 6.717514421272180236, 9.000000000000007105 ) ) ;
#1481=CARTESIAN_POINT ( 'NONE',  ( 6.751237864895159646, -6.683790977649239906, 20.49886208192143400 ) ) ;
#1487=CARTESIAN_POINT ( 'NONE',  ( -10.90442828429183919, -1.727091770866654663, 11.54999999999998295 ) ) ;
#1490=CARTESIAN_POINT ( 'NONE',  ( -7.458344646081709328, 7.390897758835805575, 6.998862081921422451 ) ) ;
#1496=CARTESIAN_POINT ( 'NONE',  ( 8.464561979789474222, 4.312909747525755400, 12.90000000000002345 ) ) ;
#1505=CARTESIAN_POINT ( 'NONE',  ( -9.814260835641038128, 5.056896391392218248, 16.85113791807854611 ) ) ;
#1514=CARTESIAN_POINT ( 'NONE',  ( -7.424621202458789426, 7.424621202458724589, -3.058133128536869244E-17 ) ) ;
#1519=CARTESIAN_POINT ( 'NONE',  ( -4.967534682030703586, 9.859792900771061852, 2.151137918078574796 ) ) ;
#1520=CARTESIAN_POINT ( 'NONE',  ( -9.375578539472099848, 1.533232399700011461, 1.701137918078535094 ) ) ;
#1531=CARTESIAN_POINT ( 'NONE',  ( -4.534861676072319270, 8.900167166472121139, 12.14999999999996305 ) ) ;
#1532=CARTESIAN_POINT ( 'NONE',  ( 8.922933199037192509, -4.490180821391404287, 17.34886208192141765 ) ) ;
#1537=CARTESIAN_POINT ( 'NONE',  ( 9.383039235653818366, -1.486127417882130208, 1.200000000000034373 ) ) ;
#1545=CARTESIAN_POINT ( 'NONE',  ( 9.333916720356675967, 4.809394265263123636, 10.89886208192140771 ) ) ;
#1551=CARTESIAN_POINT ( 'NONE',  ( 9.865911304835478290, 1.562606840307950273, 13.04999999999999538 ) ) ;
#1552=CARTESIAN_POINT ( 'NONE',  ( -9.837026868206066865, 5.012215536711413399, 14.84999999999999787 ) ) ;
#1556=CARTESIAN_POINT ( 'NONE',  ( 6.717514421272239744, -6.717514421272154479, 19.50000000000001776 ) ) ;
#1561=CARTESIAN_POINT ( 'NONE',  ( 9.837026868206066865, -5.012215536711392083, 1.350000000000015188 ) ) ;
#1567=CARTESIAN_POINT ( 'NONE',  ( 9.837026868206070418, -5.012215536711391195, 4.350000000000036948 ) ) ;
#1571=CARTESIAN_POINT ( 'NONE',  ( 7.390897758835871301, -7.458344646081624063, 3.501137918078585987 ) ) ;
#1572=CARTESIAN_POINT ( 'NONE',  ( 8.877401133907127928, -4.579542530753017537, 18.35113791807858519 ) ) ;
#1576=ORIENTED_EDGE ( 'NONE', *, *, #3511, .F. ) ;
#1581=CARTESIAN_POINT ( 'NONE',  ( 7.063212654743467489, 7.063212654743559860, 18.74999999999998934 ) ) ;
#1582=CARTESIAN_POINT ( 'NONE',  ( -6.751237864895158758, 6.683790977649261222, 18.99886208192142334 ) ) ;
#1593=CARTESIAN_POINT ( 'NONE',  ( 1.689666864740335894, -10.36326688006720786, 5.798862081921429379 ) ) ;
#1600=CARTESIAN_POINT ( 'NONE',  ( -7.063212654743467489, -7.063212654743533214, 14.25000000000001421 ) ) ;
#1601=CARTESIAN_POINT ( 'NONE',  ( -1.642561882922479732, 10.37072757624895303, 18.29999999999998295 ) ) ;
#1608=CARTESIAN_POINT ( 'NONE',  ( 5.012215536711511987, -9.837026868205999364, 1.650000000000006128 ) ) ;
#1609=CARTESIAN_POINT ( 'NONE',  ( -10.37072757624895836, 1.642561882922381145, 5.700000000000038369 ) ) ;
#1614=CARTESIAN_POINT ( 'NONE',  ( -4.766900247265192014, -9.355568503977876205, 17.10000000000000497 ) ) ;
#1618=CARTESIAN_POINT ( 'NONE',  ( -4.967534682030703586, 9.859792900771061852, 5.151137918078567246 ) ) ;
#1619=CARTESIAN_POINT ( 'NONE',  ( 1.439022436064387511, -9.390499931835512015, 9.801137918078557831 ) ) ;
#1629=CARTESIAN_POINT ( 'NONE',  ( 1.562606840307832368, 9.865911304835510265, 15.44999999999997797 ) ) ;
#1630=CARTESIAN_POINT ( 'NONE',  ( -9.383039235653820143, 1.486127417882155521, 5.700000000000038369 ) ) ;
#1633=CARTESIAN_POINT ( 'NONE',  ( -8.464561979789474222, -4.312909747525729642, 2.400000000000013234 ) ) ;
#1641=CARTESIAN_POINT ( 'NONE',  ( 1.533232399700100945, -9.375578539472073203, 2.798862081921426714 ) ) ;
#1643=CARTESIAN_POINT ( 'NONE',  ( 1.677562661911645714, 10.91227292449347175, 7.448862081921427070 ) ) ;
#1649=CARTESIAN_POINT ( 'NONE',  ( 1.562606840307832146, 9.865911304835508489, 9.449999999999992184 ) ) ;
#1650=CARTESIAN_POINT ( 'NONE',  ( -10.90442828429183919, -1.727091770866654663, 14.55000000000000249 ) ) ;
#1656=CARTESIAN_POINT ( 'NONE',  ( -9.837026868206066865, 5.012215536711413399, 2.849999999999968114 ) ) ;
#1657=CARTESIAN_POINT ( 'NONE',  ( 5.012215536711511987, -9.837026868205999364, 4.650000000000026112 ) ) ;
#1665=CARTESIAN_POINT ( 'NONE',  ( -5.012215536711508435, 9.837026868206027785, 15.14999999999998614 ) ) ;
#1668=CARTESIAN_POINT ( 'NONE',  ( 1.595456901104624459, -10.37818827243065201, 3.801137918078595135 ) ) ;
#1669=CARTESIAN_POINT ( 'NONE',  ( 6.683790977649321619, -6.751237864895082375, 12.50113791807859265 ) ) ;
#1684=CARTESIAN_POINT ( 'NONE',  ( 6.717514421272239744, -6.717514421272154479, 13.50000000000001243 ) ) ;
#1685=CARTESIAN_POINT ( 'NONE',  ( 1.562606840307832368, 9.865911304835510265, 9.449999999999988631 ) ) ;
#1689=CARTESIAN_POINT ( 'NONE',  ( 4.534861676072321046, -8.900167166472098046, 4.650000000000027001 ) ) ;
#1696=CARTESIAN_POINT ( 'NONE',  ( 1.533232399700100945, -9.375578539472067874, 5.798862081921429379 ) ) ;
#1697=CARTESIAN_POINT ( 'NONE',  ( 1.689666864740335894, -10.36326688006720786, 14.79886208192143471 ) ) ;
#1703=CARTESIAN_POINT ( 'NONE',  ( -9.865911304835474738, -1.562606840307925626, 14.55000000000000604 ) ) ;
#1704=CARTESIAN_POINT ( 'NONE',  ( 7.771249796623105333, 7.842167650704658932, 10.74886208192140913 ) ) ;
#1713=CARTESIAN_POINT ( 'NONE',  ( -5.012215536711506658, 9.837026868206027785, 12.14999999999996305 ) ) ;
#1714=CARTESIAN_POINT ( 'NONE',  ( -4.766900247265192014, -9.355568503977876205, 2.099999999999990763 ) ) ;
#1719=CARTESIAN_POINT ( 'NONE',  ( 9.355568503977840678, 4.766900247265305701, 12.90000000000002345 ) ) ;
#1723=CARTESIAN_POINT ( 'NONE',  ( 9.377220287599001836, 4.724406229267492208, 11.90113791807857702 ) ) ;
#1724=CARTESIAN_POINT ( 'NONE',  ( -6.683790977649319842, 6.751237864895101026, 17.00113791807859442 ) ) ;
#1732=CARTESIAN_POINT ( 'NONE',  ( -9.383039235653820143, 1.486127417882154411, 14.69999999999999041 ) ) ;
#1733=CARTESIAN_POINT ( 'NONE',  ( 6.717514421272239744, -6.717514421272154479, 4.500000000000003553 ) ) ;
#1741=CARTESIAN_POINT ( 'NONE',  ( -9.858066664633883036, -1.612135949262833101, 9.548862081921404510 ) ) ;
#1742=CARTESIAN_POINT ( 'NONE',  ( 1.513077731352925115, 9.873755945037103743, 1.448862081921441947 ) ) ;
#1751=CARTESIAN_POINT ( 'NONE',  ( -1.689666864740335228, 10.36326688006723451, 7.298862081921430267 ) ) ;
#1757=CARTESIAN_POINT ( 'NONE',  ( 9.355568503977840678, 4.766900247265305701, 6.899999999999961275 ) ) ;
#1758=CARTESIAN_POINT ( 'NONE',  ( 1.642561882922480621, -10.37072757624891750, 7.800000000000029132 ) ) ;
#1762=CARTESIAN_POINT ( 'NONE',  ( -1.642561882922479732, 10.37072757624895303, 15.29999999999997939 ) ) ;
#1765=CARTESIAN_POINT ( 'NONE',  ( 7.842167650704563897, 7.771249796623202144, 11.75113791807857666 ) ) ;
#1766=CARTESIAN_POINT ( 'NONE',  ( 9.375578539472099848, -1.533232399699987702, 12.20113791807854398 ) ) ;
#1772=ORIENTED_EDGE ( 'NONE', *, *, #967, .F. ) ;
#1777=CARTESIAN_POINT ( 'NONE',  ( -9.873755945037078874, -1.513077731353020594, 1.551137918078593803 ) ) ;
#1778=CARTESIAN_POINT ( 'NONE',  ( -4.312909747525649706, -8.464561979789499091, 11.09999999999999787 ) ) ;
#1788=SURFACE_STYLE_FILL_AREA ( #392 ) ;
#1790=CARTESIAN_POINT ( 'NONE',  ( 8.464561979789474222, 4.312909747525755400, 0.9000000000000119016 ) ) ;
#1791=CARTESIAN_POINT ( 'NONE',  ( -1.689666864740335228, 10.36326688006722740, 13.29886208192143471 ) ) ;
#1797=CARTESIAN_POINT ( 'NONE',  ( -7.458344646081709328, 7.390897758835799358, 12.99886208192142512 ) ) ;
#1804=CARTESIAN_POINT ( 'NONE',  ( 9.837026868206066865, -5.012215536711391195, 4.350000000000036948 ) ) ;
#1805=CARTESIAN_POINT ( 'NONE',  ( -10.90442828429183919, -1.727091770866654663, 11.54999999999998295 ) ) ;
#1811=CARTESIAN_POINT ( 'NONE',  ( -10.90442828429184274, -1.727091770866655107, 14.55000000000000604 ) ) ;
#1814=CARTESIAN_POINT ( 'NONE',  ( -9.377220287598998283, -4.724406229267462898, 16.40113791807857524 ) ) ;
#1815=CARTESIAN_POINT ( 'NONE',  ( 1.776620879821457333, 10.89658364409028124, 8.451137918078549305 ) ) ;
#1827=CARTESIAN_POINT ( 'NONE',  ( 6.683790977649321619, -6.751237864895076157, 9.501137918078587319 ) ) ;
#1828=CARTESIAN_POINT ( 'NONE',  ( -1.562606840307830591, -9.865911304835488949, 4.950000000000017053 ) ) ;
#1840=CARTESIAN_POINT ( 'NONE',  ( -8.464561979789474222, -4.312909747525729642, 2.400000000000013234 ) ) ;
#1841=CARTESIAN_POINT ( 'NONE',  ( 7.027753727702739539, 7.098671581784288698, 1.748862081921432887 ) ) ;
#1843=SHAPE_REPRESENTATION ( 'small spring', ( #3995 ), #6704 ) ;
#1851=CARTESIAN_POINT ( 'NONE',  ( 8.900167166472158442, -4.534861676072213577, 16.35000000000000853 ) ) ;
#1852=CARTESIAN_POINT ( 'NONE',  ( 7.458344646081711105, -7.390897758835786036, 11.49886208192146775 ) ) ;
#1858=CARTESIAN_POINT ( 'NONE',  ( 7.806708723663831506, 7.806708723663930982, 6.749999999999960032 ) ) ;
#1859=CARTESIAN_POINT ( 'NONE',  ( 7.424621202458790314, -7.424621202458697944, 13.50000000000001243 ) ) ;
#1868=CARTESIAN_POINT ( 'NONE',  ( -1.595456901104623348, 10.37818827243067155, 14.30113791807856316 ) ) ;
#1869=CARTESIAN_POINT ( 'NONE',  ( -7.390897758835869524, 7.458344646081637386, 2.001137918078543354 ) ) ;
#1875=CARTESIAN_POINT ( 'NONE',  ( 10.90442828429183919, 1.727091770866679532, 10.05000000000002736 ) ) ;
#1883=CARTESIAN_POINT ( 'NONE',  ( 9.873755945037075321, 1.513077731353044131, 6.051137918078538291 ) ) ;
#1884=CARTESIAN_POINT ( 'NONE',  ( -9.383039235653820143, 1.486127417882154411, 14.69999999999999041 ) ) ;
#1894=CARTESIAN_POINT ( 'NONE',  ( 4.270415729527831772, 8.486213763410694000, 19.59886208192144963 ) ) ;
#1895=CARTESIAN_POINT ( 'NONE',  ( 4.579542530753127672, -8.877401133907065756, 8.648862081921430800 ) ) ;
#1902=CARTESIAN_POINT ( 'NONE',  ( 5.056896391392317724, -9.814260835640970626, 11.64886208192146988 ) ) ;
#1908=CARTESIAN_POINT ( 'NONE',  ( 1.642561882922480621, -10.37072757624892638, 4.800000000000026468 ) ) ;
#1916=CARTESIAN_POINT ( 'NONE',  ( 9.814260835641038128, -5.056896391392198709, 12.35113791807855677 ) ) ;
#1917=CARTESIAN_POINT ( 'NONE',  ( -4.809394265263009061, -9.333916720356716823, 7.101137918078564759 ) ) ;
#1921=CARTESIAN_POINT ( 'NONE',  ( -1.727091770866549414, -10.90442828429185695, 4.950000000000017053 ) ) ;
#1928=CARTESIAN_POINT ( 'NONE',  ( -9.375578539472099848, 1.533232399700011461, 1.701137918078535094 ) ) ;
#1929=CARTESIAN_POINT ( 'NONE',  ( 8.900167166472154889, -4.534861676072210912, 13.34999999999998188 ) ) ;
#1940=CARTESIAN_POINT ( 'NONE',  ( -4.579542530753125895, 8.877401133907090625, 19.14886208192144679 ) ) ;
#1941=CARTESIAN_POINT ( 'NONE',  ( 8.922933199037192509, -4.490180821391404287, 5.348862081921449629 ) ) ;
#1955=CARTESIAN_POINT ( 'NONE',  ( -10.37818827243067688, 1.595456901104525205, 3.698862081921452827 ) ) ;
#1963=CARTESIAN_POINT ( 'NONE',  ( -4.579542530753125895, 8.877401133907083519, 4.148862081921444123 ) ) ;
#1964=CARTESIAN_POINT ( 'NONE',  ( 7.806708723663831506, 7.806708723663931870, 3.749999999999997335 ) ) ;
#1965=CARTESIAN_POINT ( 'NONE',  ( 7.390897758835871301, -7.458344646081617846, 6.501137918078588207 ) ) ;
#1970=CARTESIAN_POINT ( 'NONE',  ( 1.642561882922480621, -10.37072757624892638, 4.800000000000026468 ) ) ;
#1976=CARTESIAN_POINT ( 'NONE',  ( -1.612135949262737844, -9.858066664633888365, 6.951137918078597266 ) ) ;
#1977=CARTESIAN_POINT ( 'NONE',  ( -4.312909747525649706, -8.464561979789507973, 17.10000000000000497 ) ) ;
#1990=CARTESIAN_POINT ( 'NONE',  ( -7.027753727702738651, -7.098671581784262941, 18.24886208192143044 ) ) ;
#1991=CARTESIAN_POINT ( 'NONE',  ( 8.442910196168311288, 4.355403765523574222, 4.898862081921403266 ) ) ;
#2008=CARTESIAN_POINT ( 'NONE',  ( 4.724406229267374968, 9.377220287599055126, 1.598862081921434308 ) ) ;
#2009=PRODUCT_CONTEXT ( 'NONE', #2233, 'mechanical' ) ;
#2013=CARTESIAN_POINT ( 'NONE',  ( 10.37072757624895836, -1.642561882922355831, 19.19999999999999574 ) ) ;
#2015=CARTESIAN_POINT ( 'NONE',  ( 4.270415729527831772, 8.486213763410688671, 4.598862081921435419 ) ) ;
#2016=CARTESIAN_POINT ( 'NONE',  ( 1.727091770866550968, 10.90442828429187294, 3.450000000000006839 ) ) ;
#2017=CARTESIAN_POINT ( 'NONE',  ( -9.377220287598998283, -4.724406229267460233, 7.401137918078573463 ) ) ;
#2020=CARTESIAN_POINT ( 'NONE',  ( 1.727091770866550968, 10.90442828429186761, 6.449999999999969091 ) ) ;
#2025=CARTESIAN_POINT ( 'NONE',  ( -9.873755945037078874, -1.513077731353020594, 16.55113791807855605 ) ) ;
#2026=CARTESIAN_POINT ( 'NONE',  ( -1.486127417882243895, 9.383039235653816590, 12.29999999999997762 ) ) ;
#2039=CARTESIAN_POINT ( 'NONE',  ( 7.063212654743467489, 7.063212654743557195, 6.749999999999960032 ) ) ;
#2040=CARTESIAN_POINT ( 'NONE',  ( -1.533232399700100057, 9.375578539472098072, 7.298862081921430267 ) ) ;
#2042=CARTESIAN_POINT ( 'NONE',  ( 9.355568503977840678, 4.766900247265305701, 9.900000000000019895 ) ) ;
#2053=CARTESIAN_POINT ( 'NONE',  ( -10.37072757624895836, 1.642561882922380923, 17.69999999999999218 ) ) ;
#2057=CARTESIAN_POINT ( 'NONE',  ( -5.056896391392315948, 9.814260835640991942, 4.148862081921444123 ) ) ;
#2066=CARTESIAN_POINT ( 'NONE',  ( 8.922933199037192509, -4.490180821391407839, 2.348862081921457623 ) ) ;
#2068=CARTESIAN_POINT ( 'NONE',  ( -9.837026868206066865, 5.012215536711413399, 2.849999999999968114 ) ) ;
#2069=CARTESIAN_POINT ( 'NONE',  ( 10.36326688006723984, -1.689666864740212215, 15.20113791807854575 ) ) ;
#2072=CARTESIAN_POINT ( 'NONE',  ( -7.424621202458789426, 7.424621202458724589, 6.000000000000005329 ) ) ;
#2079=CARTESIAN_POINT ( 'NONE',  ( 4.355403765523470305, 8.442910196168364578, 11.60113791807856742 ) ) ;
#2080=CARTESIAN_POINT ( 'NONE',  ( -6.683790977649319842, 6.751237864895101026, 5.001137918078545574 ) ) ;
#2089=CARTESIAN_POINT ( 'NONE',  ( -9.837026868206066865, 5.012215536711413399, 2.849999999999968114 ) ) ;
#2090=CARTESIAN_POINT ( 'NONE',  ( -8.900167166472156666, 4.534861676072234893, 5.849999999999989875 ) ) ;
#2091=CARTESIAN_POINT ( 'NONE',  ( -9.858066664633883036, -1.612135949262833101, 9.548862081921404510 ) ) ;
#2092=CARTESIAN_POINT ( 'NONE',  ( 9.837026868206066865, -5.012215536711392083, 19.34999999999996945 ) ) ;
#2104=CARTESIAN_POINT ( 'NONE',  ( 9.837026868206066865, -5.012215536711392083, 13.34999999999998188 ) ) ;
#2109=CARTESIAN_POINT ( 'NONE',  ( 9.333916720356675967, 4.809394265263123636, 1.898862081921442790 ) ) ;
#2120=CARTESIAN_POINT ( 'NONE',  ( 10.89658364409024749, 1.776620879821585897, 20.04886208192142050 ) ) ;
#2122=CARTESIAN_POINT ( 'NONE',  ( 9.355568503977840678, 4.766900247265305701, 9.900000000000019895 ) ) ;
#2123=CARTESIAN_POINT ( 'NONE',  ( 9.377220287599001836, 4.724406229267492208, 11.90113791807857702 ) ) ;
#2127=CARTESIAN_POINT ( 'NONE',  ( -1.642561882922479732, 10.37072757624895303, 15.29999999999997939 ) ) ;
#2129=CARTESIAN_POINT ( 'NONE',  ( -1.727091770866549414, -10.90442828429184630, 7.950000000000040146 ) ) ;
#2133=CARTESIAN_POINT ( 'NONE',  ( -4.967534682030703586, 9.859792900771061852, -0.8488620819214613977 ) ) ;
#2134=CARTESIAN_POINT ( 'NONE',  ( 9.873755945037075321, 1.513077731353044131, 6.051137918078538291 ) ) ;
#2146=CARTESIAN_POINT ( 'NONE',  ( -9.865911304835474738, -1.562606840307925626, 8.549999999999963407 ) ) ;
#2147=CARTESIAN_POINT ( 'NONE',  ( 6.717514421272239744, -6.717514421272154479, 1.500000000000001332 ) ) ;
#2148=CARTESIAN_POINT ( 'NONE',  ( 1.642561882922480621, -10.37072757624891750, 10.80000000000003268 ) ) ;
#2159=CARTESIAN_POINT ( 'NONE',  ( -7.806708723663830618, -7.806708723663901672, 17.25000000000003553 ) ) ;
#2166=CARTESIAN_POINT ( 'NONE',  ( -1.727091770866549414, -10.90442828429184630, 13.95000000000002593 ) ) ;
#2181=CARTESIAN_POINT ( 'NONE',  ( 7.458344646081711105, -7.390897758835778930, 17.49886208192142689 ) ) ;
#2183=CARTESIAN_POINT ( 'NONE',  ( -4.766900247265192014, -9.355568503977876205, 5.099999999999993427 ) ) ;
#2184=CARTESIAN_POINT ( 'NONE',  ( 7.390897758835871301, -7.458344646081617846, 18.50113791807859087 ) ) ;
#2187=CARTESIAN_POINT ( 'NONE',  ( 5.012215536711512875, -9.837026868206002916, 1.650000000000006128 ) ) ;
#2190=CARTESIAN_POINT ( 'NONE',  ( 9.814260835641038128, -5.056896391392198709, 0.3511379180785880183 ) ) ;
#2191=CARTESIAN_POINT ( 'NONE',  ( 9.375578539472099848, -1.533232399699986370, 9.201137918078538647 ) ) ;
#2203=CARTESIAN_POINT ( 'NONE',  ( -9.383039235653820143, 1.486127417882154411, 11.69999999999998863 ) ) ;
#2204=CARTESIAN_POINT ( 'NONE',  ( 9.858066664633883036, 1.612135949262857526, 20.04886208192142050 ) ) ;
#2213=CARTESIAN_POINT ( 'NONE',  ( 1.642561882922480621, -10.37072757624891750, 10.80000000000003268 ) ) ;
#2216=CARTESIAN_POINT ( 'NONE',  ( 7.458344646081711105, -7.390897758835778930, 8.498862081921462419 ) ) ;
#2221=CARTESIAN_POINT ( 'NONE',  ( 4.534861676072321046, -8.900167166472096270, 7.649999999999992362 ) ) ;
#2227=CARTESIAN_POINT ( 'NONE',  ( -4.579542530753125895, 8.877401133907090625, 10.14886208192142725 ) ) ;
#2230=CARTESIAN_POINT ( 'NONE',  ( -10.36326688006724162, 1.689666864740236862, 10.70113791807854220 ) ) ;
#2233=APPLICATION_CONTEXT ( 'automotive_design' ) ;
#2234=CARTESIAN_POINT ( 'NONE',  ( 10.90442828429184274, 1.727091770866679310, 1.049999999999966738 ) ) ;
#2237=CARTESIAN_POINT ( 'NONE',  ( 4.355403765523470305, 8.442910196168369907, 14.60113791807856920 ) ) ;
#2238=CARTESIAN_POINT ( 'NONE',  ( -9.375578539472099848, 1.533232399700011461, 4.701137918078535982 ) ) ;
#2249=CARTESIAN_POINT ( 'NONE',  ( -7.063212654743466601, -7.063212654743534991, 8.250000000000028422 ) ) ;
#2250=CARTESIAN_POINT ( 'NONE',  ( 8.442910196168311288, 4.355403765523576887, 16.89886208192141126 ) ) ;
#2251=EDGE_CURVE ( 'NONE', #879, #8995, #3817, .T. ) ;
#2257=CARTESIAN_POINT ( 'NONE',  ( 10.37072757624895836, -1.642561882922356498, 13.19999999999998863 ) ) ;
#2261=CARTESIAN_POINT ( 'NONE',  ( -1.689666864740335228, 10.36326688006722740, 13.29886208192143471 ) ) ;
#2267=CARTESIAN_POINT ( 'NONE',  ( -7.063212654743467489, -7.063212654743533214, 11.24999999999999467 ) ) ;
#2275=CARTESIAN_POINT ( 'NONE',  ( 9.390499931835536884, -1.439022436064273158, 8.198862081921454603 ) ) ;
#2277=CARTESIAN_POINT ( 'NONE',  ( -9.355568503977838901, -4.766900247265280832, 2.400000000000013234 ) ) ;
#2278=CARTESIAN_POINT ( 'NONE',  ( -7.842167650704559456, -7.771249796623180828, 13.25113791807857311 ) ) ;
#2284=CARTESIAN_POINT ( 'NONE',  ( 10.37072757624895836, -1.642561882922355609, 4.199999999999981526 ) ) ;
#2290=CARTESIAN_POINT ( 'NONE',  ( 9.814260835641038128, -5.056896391392198709, 9.351137918078563871 ) ) ;
#2291=CARTESIAN_POINT ( 'NONE',  ( -7.098671581784199880, -7.027753727702804376, 7.251137918078588207 ) ) ;
#2302=CARTESIAN_POINT ( 'NONE',  ( 4.490180821391514421, -8.922933199037132113, 0.6511379180785785703 ) ) ;
#2303=CARTESIAN_POINT ( 'NONE',  ( 7.027753727702739539, 7.098671581784288698, 19.74886208192143044 ) ) ;
#2304=DIRECTION ( 'NONE',  ( 0.7063021515967560227, 0.7063021515967630171, 0.04769215134145720486 ) ) ;
#2313=CARTESIAN_POINT ( 'NONE',  ( -9.859792900771106261, 4.967534682030606774, 6.848862081921402556 ) ) ;
#2317=CARTESIAN_POINT ( 'NONE',  ( -6.717514421272238856, 6.717514421272181124, 6.000000000000005329 ) ) ;
#2318=CARTESIAN_POINT ( 'NONE',  ( 7.806708723663831506, 7.806708723663930982, 12.75000000000000533 ) ) ;
#2329=FACE_OUTER_BOUND ( 'NONE', #3355, .T. ) ;
#2330=CARTESIAN_POINT ( 'NONE',  ( -7.424621202458789426, 7.424621202458723701, 9.000000000000007105 ) ) ;
#2338=CARTESIAN_POINT ( 'NONE',  ( 9.814260835641038128, -5.056896391392198709, 3.351137918078579858 ) ) ;
#2339=CARTESIAN_POINT ( 'NONE',  ( 7.098671581784200768, 7.027753727702831021, 17.75113791807856245 ) ) ;
#2351=CARTESIAN_POINT ( 'NONE',  ( 6.717514421272239744, -6.717514421272154479, 16.50000000000001421 ) ) ;
#2352=CARTESIAN_POINT ( 'NONE',  ( -9.390499931835536884, 1.439022436064298249, 15.69886208192145816 ) ) ;
#2361=CARTESIAN_POINT ( 'NONE',  ( -1.689666864740335228, 10.36326688006723451, 7.298862081921430267 ) ) ;
#2367=CARTESIAN_POINT ( 'NONE',  ( 1.486127417882244783, -9.383039235653791721, 13.80000000000003446 ) ) ;
#2368=CARTESIAN_POINT ( 'NONE',  ( 10.90442828429183919, 1.727091770866679532, 19.04999999999997939 ) ) ;
#2376=CARTESIAN_POINT ( 'NONE',  ( 9.355568503977840678, 4.766900247265305701, 0.9000000000000119016 ) ) ;
#2377=CARTESIAN_POINT ( 'NONE',  ( 7.806708723663831506, 7.806708723663925653, 9.749999999999982236 ) ) ;
#2384=CARTESIAN_POINT ( 'NONE',  ( 1.642561882922480621, -10.37072757624892638, 16.80000000000003624 ) ) ;
#2387=CARTESIAN_POINT ( 'NONE',  ( 10.91227292449344155, 1.677562661911773390, 3.051137918078546285 ) ) ;
#2388=CARTESIAN_POINT ( 'NONE',  ( -1.612135949262737844, -9.858066664633888365, 9.951137918078590161 ) ) ;
#2399=CARTESIAN_POINT ( 'NONE',  ( 8.464561979789474222, 4.312909747525755400, 18.90000000000002700 ) ) ;
#2400=CARTESIAN_POINT ( 'NONE',  ( -6.717514421272238856, 6.717514421272180236, 9.000000000000007105 ) ) ;
#2411=CARTESIAN_POINT ( 'NONE',  ( 8.922933199037192509, -4.490180821391407839, 2.348862081921457623 ) ) ;
#2414=CARTESIAN_POINT ( 'NONE',  ( 9.859792900771104485, -4.967534682030585458, 5.348862081921449629 ) ) ;
#2419=CARTESIAN_POINT ( 'NONE',  ( 1.562606840307832146, 9.865911304835501383, 6.449999999999970868 ) ) ;
#2420=CARTESIAN_POINT ( 'NONE',  ( 7.806708723663831506, 7.806708723663925653, 15.74999999999996803 ) ) ;
#2428=CARTESIAN_POINT ( 'NONE',  ( 5.012215536711511987, -9.837026868205999364, 1.650000000000006128 ) ) ;
#2434=CARTESIAN_POINT ( 'NONE',  ( -7.806708723663831506, -7.806708723663902560, 11.24999999999999467 ) ) ;
#2436=CARTESIAN_POINT ( 'NONE',  ( -7.842167650704559456, -7.771249796623176387, 1.251137918078559563 ) ) ;
#2437=CARTESIAN_POINT ( 'NONE',  ( 9.873755945037075321, 1.513077731353043243, 15.05113791807855961 ) ) ;
#2448=CARTESIAN_POINT ( 'NONE',  ( -1.562606840307830591, -9.865911304835478290, 13.95000000000002593 ) ) ;
#2449=CARTESIAN_POINT ( 'NONE',  ( -4.534861676072319270, 8.900167166472121139, 3.149999999999957723 ) ) ;
#2452=CARTESIAN_POINT ( 'NONE',  ( 8.900167166472158442, -4.534861676072210024, 4.350000000000036948 ) ) ;
#2455=ORIENTED_EDGE ( 'NONE', *, *, #967, .T. ) ;
#2459=CARTESIAN_POINT ( 'NONE',  ( 4.579542530753127672, -8.877401133907065756, 5.648862081921440570 ) ) ;
#2460=CARTESIAN_POINT ( 'NONE',  ( 1.689666864740335894, -10.36326688006720786, 17.79886208192143471 ) ) ;
#2461=CARTESIAN_POINT ( 'NONE',  ( 7.458344646081711105, -7.390897758835778930, 14.49886208192142867 ) ) ;
#2467=CARTESIAN_POINT ( 'NONE',  ( -7.424621202458789426, 7.424621202458724589, 18.00000000000001421 ) ) ;
#2473=CARTESIAN_POINT ( 'NONE',  ( -9.837026868206066865, 5.012215536711416064, 11.84999999999997478 ) ) ;
#2474=CARTESIAN_POINT ( 'NONE',  ( 9.355568503977840678, 4.766900247265305701, 3.899999999999959055 ) ) ;
#2480=CARTESIAN_POINT ( 'NONE',  ( 10.90442828429184274, 1.727091770866679310, 16.04999999999995808 ) ) ;
#2484=CARTESIAN_POINT ( 'NONE',  ( 7.842167650704563897, 7.771249796623202144, 5.751137918078548239 ) ) ;
#2485=CARTESIAN_POINT ( 'NONE',  ( -7.098671581784199880, -7.027753727702804376, 10.25113791807858021 ) ) ;
#2500=CARTESIAN_POINT ( 'NONE',  ( 8.900167166472154889, -4.534861676072213577, 16.35000000000000497 ) ) ;
#2501=CARTESIAN_POINT ( 'NONE',  ( 8.900167166472154889, -4.534861676072210024, 10.35000000000002274 ) ) ;
#2513=CARTESIAN_POINT ( 'NONE',  ( 9.858066664633883036, 1.612135949262857082, 11.04886208192144359 ) ) ;
#2514=CARTESIAN_POINT ( 'NONE',  ( -4.579542530753125895, 8.877401133907090625, 1.148862081921408151 ) ) ;
#2521=CARTESIAN_POINT ( 'NONE',  ( 9.333916720356675967, 4.809394265263123636, 4.898862081921403266 ) ) ;
#2529=CARTESIAN_POINT ( 'NONE',  ( -5.012215536711506658, 9.837026868206022456, 6.149999999999980815 ) ) ;
#2530=CARTESIAN_POINT ( 'NONE',  ( 10.37072757624895836, -1.642561882922355609, 7.199999999999984190 ) ) ;
#2534=CARTESIAN_POINT ( 'NONE',  ( -1.727091770866549414, -10.90442828429184807, 13.95000000000002416 ) ) ;
#2539=CARTESIAN_POINT ( 'NONE',  ( -1.776620879821455556, -10.89658364409025637, 12.95113791807858128 ) ) ;
#2540=CARTESIAN_POINT ( 'NONE',  ( -1.612135949262737844, -9.858066664633888365, 12.95113791807858128 ) ) ;
#2552=CARTESIAN_POINT ( 'NONE',  ( -7.098671581784199880, -7.027753727702804376, 1.251137918078559563 ) ) ;
#2553=CARTESIAN_POINT ( 'NONE',  ( 1.486127417882244783, -9.383039235653791721, 4.800000000000026468 ) ) ;
#2563=FILL_AREA_STYLE_COLOUR ( '', #2962 ) ;
#2566=CARTESIAN_POINT ( 'NONE',  ( -7.458344646081709328, 7.390897758835805575, 15.99886208192142512 ) ) ;
#2572=CARTESIAN_POINT ( 'NONE',  ( -8.900167166472160218, 4.534861676072232228, 14.84999999999999609 ) ) ;
#2573=CARTESIAN_POINT ( 'NONE',  ( 10.37818827243067510, -1.595456901104499448, 11.19886208192145816 ) ) ;
#2577=FACE_OUTER_BOUND ( 'NONE', #6322, .T. ) ;
#2581=CARTESIAN_POINT ( 'NONE',  ( -9.355568503977838901, -4.766900247265279944, 5.400000000000016342 ) ) ;
#2582=CARTESIAN_POINT ( 'NONE',  ( -10.37072757624895836, 1.642561882922380923, 17.69999999999999218 ) ) ;
#2585=CARTESIAN_POINT ( 'NONE',  ( 9.837026868206070418, -5.012215536711395636, 16.35000000000000853 ) ) ;
#2588=CARTESIAN_POINT ( 'NONE',  ( -7.390897758835869524, 7.458344646081637386, 11.00113791807855002 ) ) ;
#2589=CARTESIAN_POINT ( 'NONE',  ( -4.967534682030703586, 9.859792900771061852, 8.151137918078559252 ) ) ;
#2599=CARTESIAN_POINT ( 'NONE',  ( 6.683790977649321619, -6.751237864895082375, 3.501137918078585987 ) ) ;
#2600=CARTESIAN_POINT ( 'NONE',  ( -8.464561979789474222, -4.312909747525729642, 2.400000000000013234 ) ) ;
#2601=DIRECTION ( 'NONE',  ( 0.7071067811865510144, -0.7071067811865440200, 0.000000000000000000 ) ) ;
#2609=CARTESIAN_POINT ( 'NONE',  ( 4.534861676072320158, -8.900167166472098046, 1.650000000000006128 ) ) ;
#2610=CARTESIAN_POINT ( 'NONE',  ( 4.724406229267374968, 9.377220287599064008, 16.59886208192139989 ) ) ;
#2618=CARTESIAN_POINT ( 'NONE',  ( -5.056896391392315948, 9.814260835640997271, 7.148862081921437017 ) ) ;
#2624=CARTESIAN_POINT ( 'NONE',  ( -1.727091770866549414, -10.90442828429185695, 4.950000000000017053 ) ) ;
#2625=CARTESIAN_POINT ( 'NONE',  ( 5.012215536711511987, -9.837026868205999364, 16.64999999999999858 ) ) ;
#2633=CARTESIAN_POINT ( 'NONE',  ( 4.809394265263009061, 9.333916720356734587, 11.60113791807856742 ) ) ;
#2634=CARTESIAN_POINT ( 'NONE',  ( 7.390897758835871301, -7.458344646081618734, 0.5011379180785839882 ) ) ;
#2639=CARTESIAN_POINT ( 'NONE',  ( -4.766900247265192014, -9.355568503977867323, 11.09999999999999787 ) ) ;
#2648=CARTESIAN_POINT ( 'NONE',  ( 9.375578539472099848, -1.533232399699987702, 3.201137918078536426 ) ) ;
#2649=CARTESIAN_POINT ( 'NONE',  ( 8.900167166472154889, -4.534861676072210912, 19.34999999999996945 ) ) ;
#2660=CARTESIAN_POINT ( 'NONE',  ( -1.513077731352923339, -9.873755945037078874, 17.94886208192144395 ) ) ;
#2661=CARTESIAN_POINT ( 'NONE',  ( 1.513077731352925115, 9.873755945037103743, 7.448862081921427070 ) ) ;
#2663=UNCERTAINTY_MEASURE_WITH_UNIT (LENGTH_MEASURE( 1.000000000000000082E-05 ), #102, 'distance_accuracy_value', 'NONE');
#2670=CARTESIAN_POINT ( 'NONE',  ( -4.724406229267374968, -9.377220287599046245, 12.09886208192144252 ) ) ;
#2676=CARTESIAN_POINT ( 'NONE',  ( 9.355568503977840678, 4.766900247265305701, 9.900000000000019895 ) ) ;
#2686=CARTESIAN_POINT ( 'NONE',  ( -9.814260835641038128, 5.056896391392221801, 13.85113791807855321 ) ) ;
#2687=CARTESIAN_POINT ( 'NONE',  ( -1.776620879821455556, -10.89658364409025637, 6.951137918078597266 ) ) ;
#2693=CARTESIAN_POINT ( 'NONE',  ( 9.355568503977840678, 4.766900247265305701, 3.899999999999959055 ) ) ;
#2700=CARTESIAN_POINT ( 'NONE',  ( 1.612135949262739398, 9.858066664633913234, 5.451137918078557298 ) ) ;
#2701=CARTESIAN_POINT ( 'NONE',  ( 7.098671581784200768, 7.027753727702831021, -0.2488620819214366897 ) ) ;
#2709=CARTESIAN_POINT ( 'NONE',  ( -4.270415729527831772, -8.486213763410670907, 18.09886208192144252 ) ) ;
#2710=CARTESIAN_POINT ( 'NONE',  ( -9.858066664633883036, -1.612135949262831547, 6.548862081921412504 ) ) ;
#2717=CARTESIAN_POINT ( 'NONE',  ( -10.89658364409024749, -1.776620879821561472, 9.548862081921404510 ) ) ;
#2724=CARTESIAN_POINT ( 'NONE',  ( -9.837026868206066865, 5.012215536711416064, 17.85000000000001918 ) ) ;
#2730=CARTESIAN_POINT ( 'NONE',  ( -6.751237864895158758, 6.683790977649255005, 3.998862081921419342 ) ) ;
#2732=CARTESIAN_POINT ( 'NONE',  ( -10.36326688006724162, 1.689666864740235308, 16.70113791807854398 ) ) ;
#2733=CARTESIAN_POINT ( 'NONE',  ( 10.36326688006723984, -1.689666864740210883, 6.201137918078538647 ) ) ;
#2738=CARTESIAN_POINT ( 'NONE',  ( 1.727091770866550968, 10.90442828429187294, 12.44999999999995666 ) ) ;
#2744=CARTESIAN_POINT ( 'NONE',  ( -9.873755945037078874, -1.513077731353020594, 7.551137918078578259 ) ) ;
#2745=CARTESIAN_POINT ( 'NONE',  ( -1.562606840307830591, -9.865911304835478290, 16.94999999999998863 ) ) ;
#2756=CARTESIAN_POINT ( 'NONE',  ( 9.390499931835536884, -1.439022436064273158, 14.19886208192146171 ) ) ;
#2757=CARTESIAN_POINT ( 'NONE',  ( -9.390499931835536884, 1.439022436064298249, 3.698862081921452827 ) ) ;
#2772=CARTESIAN_POINT ( 'NONE',  ( -7.458344646081709328, 7.390897758835799358, 3.998862081921419342 ) ) ;
#2780=CARTESIAN_POINT ( 'NONE',  ( 9.333916720356675967, 4.809394265263123636, 19.89886208192141481 ) ) ;
#2782=CARTESIAN_POINT ( 'NONE',  ( -1.642561882922479732, 10.37072757624895303, 3.299999999999969624 ) ) ;
#2783=CARTESIAN_POINT ( 'NONE',  ( 1.595456901104624459, -10.37818827243064490, 6.801137918078597799 ) ) ;
#2786=CARTESIAN_POINT ( 'NONE',  ( -10.37072757624895836, 1.642561882922380034, 11.69999999999998863 ) ) ;
#2793=CARTESIAN_POINT ( 'NONE',  ( -8.877401133907129704, 4.579542530753038854, 16.85113791807854611 ) ) ;
#2794=CARTESIAN_POINT ( 'NONE',  ( -8.464561979789474222, -4.312909747525728754, 17.39999999999997016 ) ) ;
#2810=CARTESIAN_POINT ( 'NONE',  ( 7.063212654743467489, 7.063212654743557195, 0.7499999999999762412 ) ) ;
#2811=CARTESIAN_POINT ( 'NONE',  ( 6.751237864895159646, -6.683790977649239906, 11.49886208192146775 ) ) ;
#2813=CARTESIAN_POINT ( 'NONE',  ( 9.837026868206066865, -5.012215536711391195, 10.35000000000002274 ) ) ;
#2823=CARTESIAN_POINT ( 'NONE',  ( 4.766900247265192903, 9.355568503977902850, 15.60000000000000320 ) ) ;
#2827=CARTESIAN_POINT ( 'NONE',  ( -9.333916720356675967, -4.809394265263095214, 3.398862081921444123 ) ) ;
#2836=CARTESIAN_POINT ( 'NONE',  ( 9.859792900771104485, -4.967534682030585458, 17.34886208192141765 ) ) ;
#2838=CARTESIAN_POINT ( 'NONE',  ( 7.424621202458790314, -7.424621202458697944, 7.500000000000007105 ) ) ;
#2839=CARTESIAN_POINT ( 'NONE',  ( 7.390897758835871301, -7.458344646081624063, 12.50113791807859265 ) ) ;
#2843=CARTESIAN_POINT ( 'NONE',  ( -1.642561882922479732, 10.37072757624896191, 9.299999999999975842 ) ) ;
#2849=CARTESIAN_POINT ( 'NONE',  ( 9.873755945037075321, 1.513077731353043243, 15.05113791807855961 ) ) ;
#2850=CARTESIAN_POINT ( 'NONE',  ( 7.063212654743467489, 7.063212654743557195, 12.75000000000000533 ) ) ;
#2854=EDGE_LOOP ( 'NONE', ( #4126, #5157 ) ) ;
#2861=CARTESIAN_POINT ( 'NONE',  ( 1.562606840307832368, 9.865911304835503159, 6.449999999999969091 ) ) ;
#2862=CARTESIAN_POINT ( 'NONE',  ( -7.027753727702738651, -7.098671581784262941, 12.24886208192144998 ) ) ;
#2863=CARTESIAN_POINT ( 'NONE',  ( 1.727091770866550968, 10.90442828429187294, 15.44999999999997797 ) ) ;
#2873=CARTESIAN_POINT ( 'NONE',  ( 1.642561882922480621, -10.37072757624892638, 16.80000000000003624 ) ) ;
#2878=CARTESIAN_POINT ( 'NONE',  ( -5.012215536711506658, 9.837026868206027785, 15.14999999999998259 ) ) ;
#2887=CARTESIAN_POINT ( 'NONE',  ( 4.724406229267374968, 9.377220287599064008, 16.59886208192139989 ) ) ;
#2888=CARTESIAN_POINT ( 'NONE',  ( 1.727091770866550968, 10.90442828429187294, 9.449999999999988631 ) ) ;
#2889=CARTESIAN_POINT ( 'NONE',  ( -1.595456901104623348, 10.37818827243066622, 11.30113791807855961 ) ) ;
#2893=CARTESIAN_POINT ( 'NONE',  ( 9.859792900771104485, -4.967534682030589011, 2.348862081921457623 ) ) ;
#2898=CARTESIAN_POINT ( 'NONE',  ( -9.873755945037078874, -1.513077731353019706, 10.55113791807857204 ) ) ;
#2899=CARTESIAN_POINT ( 'NONE',  ( 1.439022436064387511, -9.390499931835512015, 0.8011379180785925813 ) ) ;
#2910=CARTESIAN_POINT ( 'NONE',  ( 9.355568503977840678, 4.766900247265305701, 0.9000000000000119016 ) ) ;
#2911=CARTESIAN_POINT ( 'NONE',  ( 9.865911304835474738, 1.562606840307948719, 4.049999999999988276 ) ) ;
#2912=CARTESIAN_POINT ( 'NONE',  ( 4.270415729527831772, 8.486213763410694000, 19.59886208192144963 ) ) ;
#2913=CARTESIAN_POINT ( 'NONE',  ( 10.37072757624895836, -1.642561882922356498, 13.19999999999998863 ) ) ;
#2923=CARTESIAN_POINT ( 'NONE',  ( -9.837026868206066865, 5.012215536711413399, 14.84999999999999787 ) ) ;
#2926=COLOUR_RGB ( '', 0.31764706, 0.68627451, 0.89019608) ;
#2928=CARTESIAN_POINT ( 'NONE',  ( 10.37072757624895836, -1.642561882922356498, 16.19999999999999218 ) ) ;
#2939=CARTESIAN_POINT ( 'NONE',  ( -7.458344646081709328, 7.390897758835805575, 15.99886208192142512 ) ) ;
#2941=CARTESIAN_POINT ( 'NONE',  ( 10.90442828429183919, 1.727091770866679532, 1.049999999999966738 ) ) ;
#2942=CARTESIAN_POINT ( 'NONE',  ( 10.91227292449344155, 1.677562661911773167, 18.05113791807859513 ) ) ;
#2948=CARTESIAN_POINT ( 'NONE',  ( 7.424621202458790314, -7.424621202458697944, 1.500000000000001332 ) ) ;
#2951=CARTESIAN_POINT ( 'NONE',  ( 10.91227292449344155, 1.677562661911773390, 0.05113791807855379290 ) ) ;
#2952=CARTESIAN_POINT ( 'NONE',  ( -4.355403765523468529, -8.442910196168346815, 7.101137918078564759 ) ) ;
#2962=COLOUR_RGB ( '', 0.31764706, 0.68627451, 0.89019608) ;
#2963=CARTESIAN_POINT ( 'NONE',  ( 5.012215536711511987, -9.837026868205999364, 1.650000000000006128 ) ) ;
#2964=CARTESIAN_POINT ( 'NONE',  ( -8.464561979789474222, -4.312909747525728754, 11.39999999999996660 ) ) ;
#2965=CARTESIAN_POINT ( 'NONE',  ( -4.579542530753125895, 8.877401133907090625, 16.14886208192145389 ) ) ;
#2975=CARTESIAN_POINT ( 'NONE',  ( 7.424621202458790314, -7.424621202458697944, 19.50000000000001776 ) ) ;
#2982=CARTESIAN_POINT ( 'NONE',  ( 10.37818827243067510, -1.595456901104499448, 11.19886208192145816 ) ) ;
#2987=CARTESIAN_POINT ( 'NONE',  ( 8.464561979789474222, 4.312909747525755400, 6.899999999999961275 ) ) ;
#2995=CARTESIAN_POINT ( 'NONE',  ( -9.390499931835536884, 1.439022436064298249, 12.69886208192145816 ) ) ;
#2997=CARTESIAN_POINT ( 'NONE',  ( 7.424621202458790314, -7.424621202458697944, 1.500000000000001332 ) ) ;
#2998=CARTESIAN_POINT ( 'NONE',  ( 1.595456901104624459, -10.37818827243064490, 15.80113791807855961 ) ) ;
#3003=CARTESIAN_POINT ( 'NONE',  ( -4.766900247265192014, -9.355568503977876205, 2.099999999999990763 ) ) ;
#3007=CARTESIAN_POINT ( 'NONE',  ( -4.355403765523468529, -8.442910196168346815, 16.10113791807856742 ) ) ;
#3008=CARTESIAN_POINT ( 'NONE',  ( -9.873755945037078874, -1.513077731353019706, 4.551137918078585365 ) ) ;
#3021=CARTESIAN_POINT ( 'NONE',  ( -9.383039235653820143, 1.486127417882155521, 5.700000000000038369 ) ) ;
#3022=CARTESIAN_POINT ( 'NONE',  ( 9.858066664633883036, 1.612135949262857526, 17.04886208192142760 ) ) ;
#3030=CARTESIAN_POINT ( 'NONE',  ( 5.012215536711511987, -9.837026868205999364, 13.65000000000003233 ) ) ;
#3034=CARTESIAN_POINT ( 'NONE',  ( -5.056896391392315948, 9.814260835640991942, 13.14886208192146633 ) ) ;
#3040=CARTESIAN_POINT ( 'NONE',  ( -8.900167166472160218, 4.534861676072235781, 11.84999999999997478 ) ) ;
#3046=CARTESIAN_POINT ( 'NONE',  ( -6.751237864895158758, 6.683790977649255005, 12.99886208192142512 ) ) ;
#3048=CARTESIAN_POINT ( 'NONE',  ( 1.727091770866550968, 10.90442828429187294, 0.4499999999999856337 ) ) ;
#3049=CARTESIAN_POINT ( 'NONE',  ( 4.809394265263009061, 9.333916720356739916, 14.60113791807856920 ) ) ;
#3053=CARTESIAN_POINT ( 'NONE',  ( -5.012215536711508435, 9.837026868206027785, 3.149999999999958611 ) ) ;
#3057=CARTESIAN_POINT ( 'NONE',  ( 10.91227292449344155, 1.677562661911774944, 9.051137918078573819 ) ) ;
#3058=CARTESIAN_POINT ( 'NONE',  ( -4.355403765523468529, -8.442910196168352144, 4.101137918078561206 ) ) ;
#3070=CARTESIAN_POINT ( 'NONE',  ( 8.877401133907127928, -4.579542530753017537, 0.3511379180785880183 ) ) ;
#3071=CARTESIAN_POINT ( 'NONE',  ( 7.027753727702739539, 7.098671581784283369, 13.74886208192144643 ) ) ;
#3083=CARTESIAN_POINT ( 'NONE',  ( 5.056896391392317724, -9.814260835640970626, 8.648862081921430800 ) ) ;
#3088=CARTESIAN_POINT ( 'NONE',  ( -9.383039235653820143, 1.486127417882155521, 5.700000000000038369 ) ) ;
#3090=CARTESIAN_POINT ( 'NONE',  ( -7.806708723663830618, -7.806708723663901672, 17.25000000000003553 ) ) ;
#3097=CARTESIAN_POINT ( 'NONE',  ( 1.513077731352925115, 9.873755945037100190, 13.44886208192141197 ) ) ;
#3100=CARTESIAN_POINT ( 'NONE',  ( 7.806708723663831506, 7.806708723663931870, 3.749999999999997335 ) ) ;
#3106=CARTESIAN_POINT ( 'NONE',  ( -9.355568503977838901, -4.766900247265279944, 5.400000000000016342 ) ) ;
#3110=CARTESIAN_POINT ( 'NONE',  ( -1.776620879821455556, -10.89658364409025637, 0.9511379180785689558 ) ) ;
#3111=CARTESIAN_POINT ( 'NONE',  ( -1.439022436064386845, 9.390499931835535108, 8.301137918078554279 ) ) ;
#3119=CARTESIAN_POINT ( 'NONE',  ( 1.439022436064387511, -9.390499931835512015, 0.8011379180785925813 ) ) ;
#3120=CARTESIAN_POINT ( 'NONE',  ( 9.383039235653818366, -1.486127417882130208, 1.200000000000034373 ) ) ;
#3131=CARTESIAN_POINT ( 'NONE',  ( 1.689666864740335894, -10.36326688006721497, 11.79886208192143471 ) ) ;
#3136=CARTESIAN_POINT ( 'NONE',  ( 6.717514421272239744, -6.717514421272154479, 13.50000000000001243 ) ) ;
#3137=CARTESIAN_POINT ( 'NONE',  ( -1.677562661911643938, -10.91227292449344688, 2.948862081921438616 ) ) ;
#3141=ORIENTED_EDGE ( 'NONE', *, *, #2251, .T. ) ;
#3144=CARTESIAN_POINT ( 'NONE',  ( -6.717514421272238856, 6.717514421272181124, 0.000000000000000000 ) ) ;
#3150=CARTESIAN_POINT ( 'NONE',  ( 1.727091770866550968, 10.90442828429186761, 6.449999999999969091 ) ) ;
#3158=CARTESIAN_POINT ( 'NONE',  ( -7.806708723663831506, -7.806708723663907001, 8.250000000000030198 ) ) ;
#3163=CARTESIAN_POINT ( 'NONE',  ( 10.36326688006723984, -1.689666864740210883, 6.201137918078538647 ) ) ;
#3164=CARTESIAN_POINT ( 'NONE',  ( 1.776620879821457333, 10.89658364409028124, -0.5488620819214271584 ) ) ;
#3177=CARTESIAN_POINT ( 'NONE',  ( -6.717514421272238856, 6.717514421272181124, 18.00000000000001421 ) ) ;
#3178=CARTESIAN_POINT ( 'NONE',  ( 9.383039235653818366, -1.486127417882129986, 4.199999999999981526 ) ) ;
#3191=CARTESIAN_POINT ( 'NONE',  ( -1.689666864740335228, 10.36326688006722740, 4.298862081921427603 ) ) ;
#3198=CARTESIAN_POINT ( 'NONE',  ( -1.562606840307830591, -9.865911304835490725, 4.950000000000017941 ) ) ;
#3199=CARTESIAN_POINT ( 'NONE',  ( 7.424621202458790314, -7.424621202458697944, 13.50000000000001243 ) ) ;
#3207=CARTESIAN_POINT ( 'NONE',  ( -4.766900247265192014, -9.355568503977876205, 2.099999999999990763 ) ) ;
#3208=CARTESIAN_POINT ( 'NONE',  ( -1.642561882922479732, 10.37072757624895303, 0.2999999999999669598 ) ) ;
#3213=CARTESIAN_POINT ( 'NONE',  ( 9.837026868206070418, -5.012215536711392083, 13.34999999999998543 ) ) ;
#3216=CARTESIAN_POINT ( 'NONE',  ( 1.595456901104624459, -10.37818827243064668, 0.8011379180785925813 ) ) ;
#3217=CARTESIAN_POINT ( 'NONE',  ( 1.612135949262739398, 9.858066664633913234, 11.45113791807854220 ) ) ;
#3226=CARTESIAN_POINT ( 'NONE',  ( 9.383039235653818366, -1.486127417882130208, 19.19999999999999574 ) ) ;
#3227=CARTESIAN_POINT ( 'NONE',  ( -8.900167166472156666, 4.534861676072231340, 8.850000000000008527 ) ) ;
#3238=CARTESIAN_POINT ( 'NONE',  ( -5.056896391392315948, 9.814260835640991942, 13.14886208192146633 ) ) ;
#3239=CARTESIAN_POINT ( 'NONE',  ( 1.689666864740335894, -10.36326688006720786, 14.79886208192143471 ) ) ;
#3246=CARTESIAN_POINT ( 'NONE',  ( 4.766900247265192903, 9.355568503977902850, 18.60000000000000497 ) ) ;
#3252=CARTESIAN_POINT ( 'NONE',  ( -9.355568503977838901, -4.766900247265279944, 11.39999999999996660 ) ) ;
#3253=CARTESIAN_POINT ( 'NONE',  ( 9.355568503977840678, 4.766900247265305701, 6.899999999999961275 ) ) ;
#3258=CARTESIAN_POINT ( 'NONE',  ( -7.424621202458789426, 7.424621202458723701, 9.000000000000007105 ) ) ;
#3261=CARTESIAN_POINT ( 'NONE',  ( 9.814260835641038128, -5.056896391392200485, 6.351137918078572753 ) ) ;
#3262=CARTESIAN_POINT ( 'NONE',  ( -9.375578539472099848, 1.533232399700010351, 16.70113791807854398 ) ) ;
#3273=CARTESIAN_POINT ( 'NONE',  ( 1.486127417882244783, -9.383039235653791721, 16.80000000000003624 ) ) ;
#3274=CARTESIAN_POINT ( 'NONE',  ( 9.865911304835474738, 1.562606840307950051, 10.05000000000002736 ) ) ;
#3285=CARTESIAN_POINT ( 'NONE',  ( 8.922933199037192509, -4.490180821391406951, 11.34886208192143364 ) ) ;
#3286=CARTESIAN_POINT ( 'NONE',  ( -7.771249796623103556, -7.842167650704634063, 18.24886208192143044 ) ) ;
#3295=CARTESIAN_POINT ( 'NONE',  ( 1.677562661911645714, 10.91227292449347175, 10.44886208192141908 ) ) ;
#3305=CARTESIAN_POINT ( 'NONE',  ( 10.90442828429183919, 1.727091770866679532, 13.04999999999999538 ) ) ;
#3306=CARTESIAN_POINT ( 'NONE',  ( 1.727091770866550968, 10.90442828429187294, 9.449999999999988631 ) ) ;
#3308=FILL_AREA_STYLE ('',( #7028 ) ) ;
#3313=CARTESIAN_POINT ( 'NONE',  ( 5.012215536711512875, -9.837026868206002916, 10.65000000000001101 ) ) ;
#3316=CARTESIAN_POINT ( 'NONE',  ( -1.595456901104623348, 10.37818827243067155, 17.30113791807856316 ) ) ;
#3317=CARTESIAN_POINT ( 'NONE',  ( -8.877401133907129704, 4.579542530753039742, 10.85113791807856209 ) ) ;
#3321=CARTESIAN_POINT ( 'NONE',  ( 6.717514421272239744, -6.717514421272154479, 19.50000000000001776 ) ) ;
#3331=CARTESIAN_POINT ( 'NONE',  ( 9.873755945037075321, 1.513077731353043243, 9.051137918078573819 ) ) ;
#3332=CARTESIAN_POINT ( 'NONE',  ( 1.486127417882244783, -9.383039235653782839, 10.80000000000003268 ) ) ;
#3335=CARTESIAN_POINT ( 'NONE',  ( -6.717514421272238856, 6.717514421272181124, 2.585396704745767526E-18 ) ) ;
#3343=CARTESIAN_POINT ( 'NONE',  ( -1.513077731352923339, -9.873755945037078874, 11.94886208192145993 ) ) ;
#3344=CARTESIAN_POINT ( 'NONE',  ( 7.771249796623105333, 7.842167650704658932, 16.74886208192143755 ) ) ;
#3351=CARTESIAN_POINT ( 'NONE',  ( 8.900167166472158442, -4.534861676072210912, 19.34999999999997300 ) ) ;
#3352=CARTESIAN_POINT ( 'NONE',  ( 4.724406229267374968, 9.377220287599064008, 7.598862081921438971 ) ) ;
#3355=EDGE_LOOP ( 'NONE', ( #2455, #6488, #5967, #1576 ) ) ;
#3359=CARTESIAN_POINT ( 'NONE',  ( -1.642561882922479732, 10.37072757624896191, 9.299999999999975842 ) ) ;
#3360=CARTESIAN_POINT ( 'NONE',  ( -7.806708723663830618, -7.806708723663901672, 17.25000000000003553 ) ) ;
#3363=CARTESIAN_POINT ( 'NONE',  ( 10.37072757624895836, -1.642561882922356498, 13.19999999999998863 ) ) ;
#3367=CARTESIAN_POINT ( 'NONE',  ( 4.967534682030706250, -9.859792900771036983, 15.65113791807858235 ) ) ;
#3368=CARTESIAN_POINT ( 'NONE',  ( 4.490180821391514421, -8.922933199037132113, 15.65113791807858235 ) ) ;
#3379=CARTESIAN_POINT ( 'NONE',  ( 8.486213763410640709, 4.270415729527940130, 2.901137918078569466 ) ) ;
#3380=CARTESIAN_POINT ( 'NONE',  ( -1.486127417882243895, 9.383039235653816590, 3.299999999999969624 ) ) ;
#3390=CARTESIAN_POINT ( 'NONE',  ( -1.562606840307830591, -9.865911304835478290, 1.949999999999996181 ) ) ;
#3391=CARTESIAN_POINT ( 'NONE',  ( 1.677562661911645714, 10.91227292449346642, 13.44886208192141197 ) ) ;
#3398=CARTESIAN_POINT ( 'NONE',  ( 1.677562661911645714, 10.91227292449346464, 4.448862081921434175 ) ) ;
#3405=CARTESIAN_POINT ( 'NONE',  ( 10.37072757624895836, -1.642561882922355609, 10.19999999999998685 ) ) ;
#3406=CARTESIAN_POINT ( 'NONE',  ( -7.424621202458789426, 7.424621202458724589, 18.00000000000001421 ) ) ;
#3413=CARTESIAN_POINT ( 'NONE',  ( -7.424621202458789426, 7.424621202458724589, 0.000000000000000000 ) ) ;
#3414=CARTESIAN_POINT ( 'NONE',  ( -9.814260835641038128, 5.056896391392221801, 7.851137918078569200 ) ) ;
#3418=CARTESIAN_POINT ( 'NONE',  ( -9.837026868206066865, 5.012215536711413399, 8.850000000000008527 ) ) ;
#3423=CARTESIAN_POINT ( 'NONE',  ( 1.439022436064387511, -9.390499931835517344, 3.801137918078595135 ) ) ;
#3424=CARTESIAN_POINT ( 'NONE',  ( -1.562606840307830591, -9.865911304835478290, 13.95000000000002593 ) ) ;
#3435=CARTESIAN_POINT ( 'NONE',  ( -9.390499931835536884, 1.439022436064298249, 15.69886208192145816 ) ) ;
#3436=CARTESIAN_POINT ( 'NONE',  ( 6.751237864895159646, -6.683790977649233689, 5.498862081921462419 ) ) ;
#3442=CARTESIAN_POINT ( 'NONE',  ( 6.717514421272239744, -6.717514421272154479, 19.50000000000001776 ) ) ;
#3443=CARTESIAN_POINT ( 'NONE',  ( 1.689666864740335894, -10.36326688006720786, 8.798862081921429379 ) ) ;
#3448=CARTESIAN_POINT ( 'NONE',  ( 10.90442828429183919, 1.727091770866678422, 4.049999999999988276 ) ) ;
#3457=CARTESIAN_POINT ( 'NONE',  ( 9.814260835641038128, -5.056896391392198709, 15.35113791807859229 ) ) ;
#3458=CARTESIAN_POINT ( 'NONE',  ( 7.390897758835871301, -7.458344646081624063, 3.501137918078585987 ) ) ;
#3466=CARTESIAN_POINT ( 'NONE',  ( -7.424621202458789426, 7.424621202458723701, 9.000000000000007105 ) ) ;
#3476=CARTESIAN_POINT ( 'NONE',  ( 4.490180821391514421, -8.922933199037132113, 9.651137918078598332 ) ) ;
#3477=CARTESIAN_POINT ( 'NONE',  ( -4.490180821391513533, 8.922933199037158758, -0.8488620819214613977 ) ) ;
#3490=PRESENTATION_STYLE_ASSIGNMENT (( #966 ) ) ;
#3492=CARTESIAN_POINT ( 'NONE',  ( -9.858066664633883036, -1.612135949262833323, 15.54886208192143293 ) ) ;
#3493=CARTESIAN_POINT ( 'NONE',  ( -1.533232399700100057, 9.375578539472094519, 10.29886208192143293 ) ) ;
#3501=CARTESIAN_POINT ( 'NONE',  ( 5.056896391392317724, -9.814260835640970626, 8.648862081921430800 ) ) ;
#3508=CARTESIAN_POINT ( 'NONE',  ( 5.012215536711511987, -9.837026868205999364, 16.64999999999999858 ) ) ;
#3511=EDGE_CURVE ( 'NONE', #1139, #879, #330, .T. ) ;
#3517=CARTESIAN_POINT ( 'NONE',  ( -9.858066664633883036, -1.612135949262833323, 3.548862081921419609 ) ) ;
#3519=CARTESIAN_POINT ( 'NONE',  ( -1.776620879821455556, -10.89658364409025637, 15.95113791807857595 ) ) ;
#3520=CARTESIAN_POINT ( 'NONE',  ( -4.809394265263009061, -9.333916720356718599, 1.101137918078559208 ) ) ;
#3527=CARTESIAN_POINT ( 'NONE',  ( -1.642561882922479732, 10.37072757624895303, 12.29999999999997762 ) ) ;
#3533=CARTESIAN_POINT ( 'NONE',  ( -4.490180821391513533, 8.922933199037158758, 5.151137918078567246 ) ) ;
#3534=CARTESIAN_POINT ( 'NONE',  ( 6.717514421272239744, -6.717514421272154479, 16.50000000000001421 ) ) ;
#3542=CARTESIAN_POINT ( 'NONE',  ( 9.390499931835536884, -1.439022436064272936, 17.19886208192146171 ) ) ;
#3543=CARTESIAN_POINT ( 'NONE',  ( 1.533232399700100945, -9.375578539472067874, 8.798862081921429379 ) ) ;
#3555=CARTESIAN_POINT ( 'NONE',  ( 9.859792900771104485, -4.967534682030589011, 2.348862081921457623 ) ) ;
#3561=CARTESIAN_POINT ( 'NONE',  ( -5.056896391392315948, 9.814260835640997271, 19.14886208192144679 ) ) ;
#3563=CARTESIAN_POINT ( 'NONE',  ( -1.642561882922479732, 10.37072757624896191, 6.299999999999972289 ) ) ;
#3564=CARTESIAN_POINT ( 'NONE',  ( -7.390897758835869524, 7.458344646081644491, 5.001137918078545574 ) ) ;
#3568=CARTESIAN_POINT ( 'NONE',  ( 1.642561882922480621, -10.37072757624891750, 10.80000000000003268 ) ) ;
#3572=CARTESIAN_POINT ( 'NONE',  ( -8.877401133907129704, 4.579542530753042406, 13.85113791807855321 ) ) ;
#3573=CARTESIAN_POINT ( 'NONE',  ( -9.865911304835474738, -1.562606840307925626, 11.54999999999998295 ) ) ;
#3585=CARTESIAN_POINT ( 'NONE',  ( 1.562606840307832368, 9.865911304835510265, 0.4499999999999856337 ) ) ;
#3586=CARTESIAN_POINT ( 'NONE',  ( 8.922933199037192509, -4.490180821391406951, 11.34886208192143364 ) ) ;
#3588=CARTESIAN_POINT ( 'NONE',  ( -4.766900247265192014, -9.355568503977867323, 11.09999999999999787 ) ) ;
#3601=CARTESIAN_POINT ( 'NONE',  ( -1.677562661911643938, -10.91227292449344688, 2.948862081921438616 ) ) ;
#3602=PRODUCT_DEFINITION_SHAPE ( 'NONE', 'NONE',  #10164 ) ;
#3610=CARTESIAN_POINT ( 'NONE',  ( -9.333916720356675967, -4.809394265263096990, 18.39886208192140771 ) ) ;
#3611=CARTESIAN_POINT ( 'NONE',  ( 9.837026868206066865, -5.012215536711392083, 1.350000000000015188 ) ) ;
#3612=CARTESIAN_POINT ( 'NONE',  ( 4.967534682030706250, -9.859792900771036983, 12.65113791807859123 ) ) ;
#3615=CARTESIAN_POINT ( 'NONE',  ( 5.012215536711511987, -9.837026868205997587, 7.649999999999992362 ) ) ;
#3621=CARTESIAN_POINT ( 'NONE',  ( -1.612135949262737844, -9.858066664633888365, 12.95113791807858128 ) ) ;
#3622=CARTESIAN_POINT ( 'NONE',  ( 1.486127417882244783, -9.383039235653791721, 13.80000000000003446 ) ) ;
#3637=CARTESIAN_POINT ( 'NONE',  ( -9.355568503977838901, -4.766900247265280832, 2.400000000000013234 ) ) ;
#3638=CARTESIAN_POINT ( 'NONE',  ( 1.486127417882244783, -9.383039235653782839, 7.800000000000029132 ) ) ;
#3639=CARTESIAN_POINT ( 'NONE',  ( -8.922933199037192509, 4.490180821391424715, 6.848862081921446077 ) ) ;
#3640=CARTESIAN_POINT ( 'NONE',  ( -5.012215536711506658, 9.837026868206022456, 18.15000000000000924 ) ) ;
#3651=CARTESIAN_POINT ( 'NONE',  ( -5.012215536711506658, 9.837026868206022456, 18.15000000000000924 ) ) ;
#3656=CARTESIAN_POINT ( 'NONE',  ( 7.806708723663831506, 7.806708723663925653, 15.74999999999996803 ) ) ;
#3668=CARTESIAN_POINT ( 'NONE',  ( -1.677562661911643938, -10.91227292449344688, 17.94886208192144395 ) ) ;
#3671=CARTESIAN_POINT ( 'NONE',  ( -7.424621202458789426, 7.424621202458723701, 9.000000000000007105 ) ) ;
#3672=CARTESIAN_POINT ( 'NONE',  ( 7.390897758835871301, -7.458344646081617846, 15.50113791807859620 ) ) ;
#3677=CARTESIAN_POINT ( 'NONE',  ( 4.766900247265192903, 9.355568503977902850, 12.59999999999999964 ) ) ;
#3683=CARTESIAN_POINT ( 'NONE',  ( 4.490180821391514421, -8.922933199037132113, 15.65113791807858235 ) ) ;
#3684=CARTESIAN_POINT ( 'NONE',  ( 1.439022436064387511, -9.390499931835517344, 3.801137918078595135 ) ) ;
#3695=CARTESIAN_POINT ( 'NONE',  ( 9.383039235653818366, -1.486127417882129986, 10.19999999999998685 ) ) ;
#3696=CARTESIAN_POINT ( 'NONE',  ( -4.579542530753125895, 8.877401133907090625, 19.14886208192144679 ) ) ;
#3697=CARTESIAN_POINT ( 'NONE',  ( -9.355568503977838901, -4.766900247265279944, 17.39999999999997016 ) ) ;
#3707=CARTESIAN_POINT ( 'NONE',  ( -7.806708723663830618, -7.806708723663901672, 11.24999999999999467 ) ) ;
#3711=CARTESIAN_POINT ( 'NONE',  ( 7.806708723663831506, 7.806708723663931870, 18.74999999999998934 ) ) ;
#3720=CARTESIAN_POINT ( 'NONE',  ( -1.533232399700100057, 9.375578539472094519, 1.298862081921425604 ) ) ;
#3722=CARTESIAN_POINT ( 'NONE',  ( 5.012215536711511987, -9.837026868205997587, 7.649999999999992362 ) ) ;
#3723=CARTESIAN_POINT ( 'NONE',  ( 4.809394265263009061, 9.333916720356739916, 17.60113791807856742 ) ) ;
#3727=CARTESIAN_POINT ( 'NONE',  ( 7.458344646081711105, -7.390897758835786036, 2.498862081921459755 ) ) ;
#3729=CARTESIAN_POINT ( 'NONE',  ( 10.90442828429184274, 1.727091770866679088, 7.050000000000010481 ) ) ;
#3733=CARTESIAN_POINT ( 'NONE',  ( 9.377220287599001836, 4.724406229267489543, -0.09886208192143307316 ) ) ;
#3734=CARTESIAN_POINT ( 'NONE',  ( 1.612135949262739398, 9.858066664633913234, 8.451137918078549305 ) ) ;
#3747=CARTESIAN_POINT ( 'NONE',  ( -1.562606840307830591, -9.865911304835478290, 10.95000000000000462 ) ) ;
#3748=CARTESIAN_POINT ( 'NONE',  ( -8.442910196168309511, -4.355403765523546689, 15.39886208192141126 ) ) ;
#3760=CARTESIAN_POINT ( 'NONE',  ( 7.424621202458790314, -7.424621202458697944, 13.50000000000001243 ) ) ;
#3764=CARTESIAN_POINT ( 'NONE',  ( 1.677562661911645714, 10.91227292449347175, 10.44886208192141908 ) ) ;
#3772=CARTESIAN_POINT ( 'NONE',  ( -1.642561882922479732, 10.37072757624896191, 6.299999999999972289 ) ) ;
#3777=CARTESIAN_POINT ( 'NONE',  ( -4.270415729527831772, -8.486213763410670907, 9.098862081921437195 ) ) ;
#3779=CARTESIAN_POINT ( 'NONE',  ( 9.837026868206066865, -5.012215536711391195, 4.350000000000036948 ) ) ;
#3780=CARTESIAN_POINT ( 'NONE',  ( 9.814260835641038128, -5.056896391392198709, 12.35113791807855677 ) ) ;
#3791=CARTESIAN_POINT ( 'NONE',  ( 8.877401133907127928, -4.579542530753017537, 15.35113791807859229 ) ) ;
#3792=CARTESIAN_POINT ( 'NONE',  ( 8.877401133907127928, -4.579542530753017537, 0.3511379180785880183 ) ) ;
#3803=CARTESIAN_POINT ( 'NONE',  ( 8.900167166472154889, -4.534861676072210024, 4.350000000000036948 ) ) ;
#3804=CARTESIAN_POINT ( 'NONE',  ( 1.533232399700100945, -9.375578539472067874, 14.79886208192143471 ) ) ;
#3814=CARTESIAN_POINT ( 'NONE',  ( -7.424621202458789426, 7.424621202458724589, 12.00000000000001066 ) ) ;
#3817=CIRCLE ( 'NONE', #8926, 0.4999999999999994449 ) ;
#3820=CARTESIAN_POINT ( 'NONE',  ( -10.37818827243067688, 1.595456901104523428, 9.698862081921454603 ) ) ;
#3824=CARTESIAN_POINT ( 'NONE',  ( 6.717514421272239744, -6.717514421272154479, 10.50000000000000888 ) ) ;
#3830=CARTESIAN_POINT ( 'NONE',  ( -8.922933199037192509, 4.490180821391428267, 12.84886208192143009 ) ) ;
#3832=CARTESIAN_POINT ( 'NONE',  ( -5.012215536711506658, 9.837026868206027785, 0.1499999999999952482 ) ) ;
#3833=CARTESIAN_POINT ( 'NONE',  ( -9.377220287598998283, -4.724406229267462898, 13.40113791807857702 ) ) ;
#3840=CARTESIAN_POINT ( 'NONE',  ( -7.806708723663831506, -7.806708723663902560, 5.250000000000008882 ) ) ;
#3844=CARTESIAN_POINT ( 'NONE',  ( -1.595456901104623348, 10.37818827243067155, 8.301137918078554279 ) ) ;
#3845=CARTESIAN_POINT ( 'NONE',  ( 9.375578539472099848, -1.533232399699987702, 3.201137918078536426 ) ) ;
#3855=CARTESIAN_POINT ( 'NONE',  ( -4.534861676072319270, 8.900167166472122915, 9.150000000000003908 ) ) ;
#3856=CARTESIAN_POINT ( 'NONE',  ( -4.534861676072319270, 8.900167166472121139, 0.1499999999999952482 ) ) ;
#3864=CARTESIAN_POINT ( 'NONE',  ( -1.727091770866549414, -10.90442828429184630, 16.94999999999998863 ) ) ;
#3866=CARTESIAN_POINT ( 'NONE',  ( -1.677562661911643938, -10.91227292449344688, 5.948862081921430622 ) ) ;
#3873=CARTESIAN_POINT ( 'NONE',  ( 9.383039235653818366, -1.486127417882129986, 10.19999999999998685 ) ) ;
#3880=CARTESIAN_POINT ( 'NONE',  ( -1.533232399700100057, 9.375578539472089190, 13.29886208192143471 ) ) ;
#3882=CARTESIAN_POINT ( 'NONE',  ( -1.642561882922479732, 10.37072757624895303, 3.299999999999969624 ) ) ;
#3883=CARTESIAN_POINT ( 'NONE',  ( -1.642561882922479732, 10.37072757624895303, 3.299999999999969624 ) ) ;
#3888=CARTESIAN_POINT ( 'NONE',  ( 7.806708723663832394, 7.806708723663931870, 3.749999999999997780 ) ) ;
#3891=CARTESIAN_POINT ( 'NONE',  ( -9.377220287598998283, -4.724406229267460233, 7.401137918078573463 ) ) ;
#3892=CARTESIAN_POINT ( 'NONE',  ( 4.355403765523470305, 8.442910196168369907, 5.601137918078562983 ) ) ;
#3903=CARTESIAN_POINT ( 'NONE',  ( 9.873755945037075321, 1.513077731353043909, 0.05113791807855379290 ) ) ;
#3904=CARTESIAN_POINT ( 'NONE',  ( 8.464561979789474222, 4.312909747525755400, 0.9000000000000119016 ) ) ;
#3912=CARTESIAN_POINT ( 'NONE',  ( 9.859792900771104485, -4.967534682030588122, 11.34886208192143364 ) ) ;
#3918=CARTESIAN_POINT ( 'NONE',  ( -7.063212654743467489, -7.063212654743535879, 8.250000000000030198 ) ) ;
#3920=CARTESIAN_POINT ( 'NONE',  ( 7.771249796623105333, 7.842167650704658932, 1.748862081921432887 ) ) ;
#3930=CARTESIAN_POINT ( 'NONE',  ( 10.37072757624895836, -1.642561882922355609, 4.199999999999981526 ) ) ;
#3937=CARTESIAN_POINT ( 'NONE',  ( -10.90442828429184274, -1.727091770866655107, 2.550000000000035794 ) ) ;
#3940=CARTESIAN_POINT ( 'NONE',  ( 4.967534682030706250, -9.859792900771036983, 0.6511379180785785703 ) ) ;
#3941=CARTESIAN_POINT ( 'NONE',  ( -1.595456901104623348, 10.37818827243067155, -0.6988620819214501623 ) ) ;
#3950=CARTESIAN_POINT ( 'NONE',  ( 8.464561979789474222, 4.312909747525755400, 12.90000000000002345 ) ) ;
#3951=CARTESIAN_POINT ( 'NONE',  ( -6.717514421272238856, 6.717514421272176683, 3.000000000000002665 ) ) ;
#3955=CARTESIAN_POINT ( 'NONE',  ( 9.865911304835478290, 1.562606840307948941, 4.049999999999988276 ) ) ;
#3959=ADVANCED_FACE ( 'NONE', ( #1346 ), #6184, .F. ) ;
#3967=CARTESIAN_POINT ( 'NONE',  ( 4.724406229267374968, 9.377220287599060455, 10.59886208192144075 ) ) ;
#3973=CARTESIAN_POINT ( 'NONE',  ( -8.900167166472160218, 4.534861676072232228, 8.850000000000010303 ) ) ;
#3974=CARTESIAN_POINT ( 'NONE',  ( -1.689666864740335228, 10.36326688006723273, 1.298862081921425604 ) ) ;
#3985=CARTESIAN_POINT ( 'NONE',  ( -1.727091770866549414, -10.90442828429185695, 4.950000000000017053 ) ) ;
#3992=CARTESIAN_POINT ( 'NONE',  ( -10.37072757624895836, 1.642561882922381145, 8.700000000000041922 ) ) ;
#3995=AXIS2_PLACEMENT_3D ( 'NONE', #245, #8930, #7419 ) ;
#3997=CARTESIAN_POINT ( 'NONE',  ( -4.967534682030703586, 9.859792900771061852, 8.151137918078559252 ) ) ;
#3998=CARTESIAN_POINT ( 'NONE',  ( -9.375578539472099848, 1.533232399700011683, 10.70113791807854220 ) ) ;
#4007=CARTESIAN_POINT ( 'NONE',  ( 4.534861676072320158, -8.900167166472098046, 16.64999999999999858 ) ) ;
#4008=CARTESIAN_POINT ( 'NONE',  ( -4.312909747525649706, -8.464561979789507973, 5.099999999999993427 ) ) ;
#4019=CARTESIAN_POINT ( 'NONE',  ( 7.771249796623105333, 7.842167650704654491, 13.74886208192144643 ) ) ;
#4022=CARTESIAN_POINT ( 'NONE',  ( 9.859792900771104485, -4.967534682030585458, 14.34886208192142831 ) ) ;
#4029=CARTESIAN_POINT ( 'NONE',  ( 7.063212654743468377, 7.063212654743558083, 6.749999999999960920 ) ) ;
#4030=CARTESIAN_POINT ( 'NONE',  ( -4.766900247265192014, -9.355568503977876205, 17.10000000000000497 ) ) ;
#4038=CARTESIAN_POINT ( 'NONE',  ( -10.90442828429183919, -1.727091770866655329, 5.549999999999999822 ) ) ;
#4042=CARTESIAN_POINT ( 'NONE',  ( -10.37072757624895836, 1.642561882922380034, 11.69999999999998863 ) ) ;
#4045=CARTESIAN_POINT ( 'NONE',  ( 10.91227292449344155, 1.677562661911773167, 6.051137918078538291 ) ) ;
#4046=CARTESIAN_POINT ( 'NONE',  ( 1.612135949262739398, 9.858066664633906129, 14.45113791807853509 ) ) ;
#4055=CARTESIAN_POINT ( 'NONE',  ( -4.534861676072319270, 8.900167166472121139, 15.14999999999998259 ) ) ;
#4056=CARTESIAN_POINT ( 'NONE',  ( -8.900167166472156666, 4.534861676072234893, 5.849999999999989875 ) ) ;
#4068=CARTESIAN_POINT ( 'NONE',  ( -1.689666864740335228, 10.36326688006723451, 16.29886208192143471 ) ) ;
#4075=CARTESIAN_POINT ( 'NONE',  ( -7.458344646081709328, 7.390897758835805575, 6.998862081921422451 ) ) ;
#4080=CARTESIAN_POINT ( 'NONE',  ( 7.806708723663831506, 7.806708723663930982, 12.75000000000000533 ) ) ;
#4081=CARTESIAN_POINT ( 'NONE',  ( 7.806708723663831506, 7.806708723663930982, 0.7499999999999762412 ) ) ;
#4087=CARTESIAN_POINT ( 'NONE',  ( -7.424621202458789426, 7.424621202458724589, 18.00000000000001421 ) ) ;
#4092=CARTESIAN_POINT ( 'NONE',  ( -9.814260835641038128, 5.056896391392218248, 16.85113791807854611 ) ) ;
#4093=CARTESIAN_POINT ( 'NONE',  ( -4.355403765523468529, -8.442910196168346815, 16.10113791807856742 ) ) ;
#4106=CARTESIAN_POINT ( 'NONE',  ( 1.562606840307832368, 9.865911304835510265, 12.44999999999995666 ) ) ;
#4107=CARTESIAN_POINT ( 'NONE',  ( -8.900167166472156666, 4.534861676072231340, 2.849999999999968114 ) ) ;
#4117=CARTESIAN_POINT ( 'NONE',  ( 1.513077731352925115, 9.873755945037103743, 7.448862081921427070 ) ) ;
#4118=CARTESIAN_POINT ( 'NONE',  ( 7.458344646081711105, -7.390897758835778930, 17.49886208192142689 ) ) ;
#4124=CARTESIAN_POINT ( 'NONE',  ( 9.865911304835478290, 1.562606840307950273, 16.04999999999995808 ) ) ;
#4125=CARTESIAN_POINT ( 'NONE',  ( -10.37818827243067688, 1.595456901104525205, 3.698862081921452827 ) ) ;
#4126=ORIENTED_EDGE ( 'NONE', *, *, #2251, .F. ) ;
#4133=CARTESIAN_POINT ( 'NONE',  ( -10.90442828429183919, -1.727091770866655329, 8.549999999999963407 ) ) ;
#4134=CARTESIAN_POINT ( 'NONE',  ( 1.642561882922480621, -10.37072757624892638, 16.80000000000003624 ) ) ;
#4140=CARTESIAN_POINT ( 'NONE',  ( 10.90442828429184274, 1.727091770866679310, 13.04999999999999538 ) ) ;
#4142=CARTESIAN_POINT ( 'NONE',  ( 9.377220287599001836, 4.724406229267489543, 17.90113791807857524 ) ) ;
#4143=CARTESIAN_POINT ( 'NONE',  ( 8.877401133907127928, -4.579542530753017537, 15.35113791807859229 ) ) ;
#4155=CARTESIAN_POINT ( 'NONE',  ( 7.098671581784200768, 7.027753727702831021, 5.751137918078548239 ) ) ;
#4156=CARTESIAN_POINT ( 'NONE',  ( -4.312909747525649706, -8.464561979789507973, 2.099999999999990763 ) ) ;
#4169=CARTESIAN_POINT ( 'NONE',  ( 9.865911304835474738, 1.562606840307950051, 1.049999999999966738 ) ) ;
#4170=CARTESIAN_POINT ( 'NONE',  ( 10.37818827243067510, -1.595456901104499448, 14.19886208192146171 ) ) ;
#4176=CARTESIAN_POINT ( 'NONE',  ( 9.383039235653818366, -1.486127417882130208, 19.19999999999999574 ) ) ;
#4177=CARTESIAN_POINT ( 'NONE',  ( -10.37818827243067688, 1.595456901104524761, 6.698862081921455491 ) ) ;
#4184=CARTESIAN_POINT ( 'NONE',  ( -9.837026868206066865, 5.012215536711416064, 5.849999999999989875 ) ) ;
#4185=CARTESIAN_POINT ( 'NONE',  ( -1.642561882922479732, 10.37072757624895303, 12.29999999999997762 ) ) ;
#4190=CARTESIAN_POINT ( 'NONE',  ( -10.37072757624895836, 1.642561882922380034, 14.69999999999999041 ) ) ;
#4194=CARTESIAN_POINT ( 'NONE',  ( 9.814260835641038128, -5.056896391392198709, 18.35113791807858519 ) ) ;
#4195=CARTESIAN_POINT ( 'NONE',  ( -1.595456901104623348, 10.37818827243067155, 5.301137918078554279 ) ) ;
#4203=CARTESIAN_POINT ( 'NONE',  ( 1.612135949262739398, 9.858066664633913234, 8.451137918078549305 ) ) ;
#4204=CARTESIAN_POINT ( 'NONE',  ( -4.534861676072319270, 8.900167166472121139, 15.14999999999998259 ) ) ;
#4211=DIRECTION ( 'NONE',  ( 0.7063021515967569108, 0.7063021515967621289, -0.04769215134145721874 ) ) ;
#4214=CARTESIAN_POINT ( 'NONE',  ( 4.579542530753127672, -8.877401133907071085, 14.64886208192141659 ) ) ;
#4215=CARTESIAN_POINT ( 'NONE',  ( 1.677562661911645714, 10.91227292449347175, 16.44886208192140131 ) ) ;
#4225=CARTESIAN_POINT ( 'NONE',  ( 4.724406229267374968, 9.377220287599055126, 4.598862081921435419 ) ) ;
#4230=CARTESIAN_POINT ( 'NONE',  ( -10.90442828429183919, -1.727091770866655329, 5.549999999999999822 ) ) ;
#4238=CARTESIAN_POINT ( 'NONE',  ( 4.766900247265192903, 9.355568503977902850, 0.5999999999999894307 ) ) ;
#4239=CARTESIAN_POINT ( 'NONE',  ( -10.36326688006724162, 1.689666864740235308, 7.701137918078540423 ) ) ;
#4245=CARTESIAN_POINT ( 'NONE',  ( -10.90442828429183919, -1.727091770866654663, 11.54999999999998295 ) ) ;
#4254=CARTESIAN_POINT ( 'NONE',  ( -8.877401133907129704, 4.579542530753042406, 4.851137918078532785 ) ) ;
#4255=CARTESIAN_POINT ( 'NONE',  ( -8.900167166472156666, 4.534861676072231340, 14.84999999999999787 ) ) ;
#4264=ADVANCED_FACE ( 'NONE', ( #2577 ), #7069, .T. ) ;
#4266=CARTESIAN_POINT ( 'NONE',  ( 8.442910196168311288, 4.355403765523574222, 19.89886208192141481 ) ) ;
#4267=CARTESIAN_POINT ( 'NONE',  ( -6.751237864895158758, 6.683790977649260334, 9.998862081921425116 ) ) ;
#4274=CARTESIAN_POINT ( 'NONE',  ( 10.37818827243067510, -1.595456901104500780, 5.198862081921453715 ) ) ;
#4280=CARTESIAN_POINT ( 'NONE',  ( 5.012215536711511987, -9.837026868205999364, 10.65000000000000924 ) ) ;
#4284=( GEOMETRIC_REPRESENTATION_CONTEXT ( 3 ) GLOBAL_UNCERTAINTY_ASSIGNED_CONTEXT ( ( #5854 ) ) GLOBAL_UNIT_ASSIGNED_CONTEXT ( ( #5086, #187, #238 ) ) REPRESENTATION_CONTEXT ( 'NONE', 'WORKASPACE' ) );
#4287=CARTESIAN_POINT ( 'NONE',  ( 1.677562661911645714, 10.91227292449347175, 16.44886208192140131 ) ) ;
#4288=CARTESIAN_POINT ( 'NONE',  ( -7.842167650704559456, -7.771249796623176387, 10.25113791807858021 ) ) ;
#4289=CARTESIAN_POINT ( 'NONE',  ( 10.36326688006723984, -1.689666864740212215, 0.2011379180785754783 ) ) ;
#4295=CARTESIAN_POINT ( 'NONE',  ( -9.355568503977838901, -4.766900247265279944, 5.400000000000016342 ) ) ;
#4302=CIRCLE ( 'NONE', #6441, 0.4999999999999994449 ) ;
#4304=CARTESIAN_POINT ( 'NONE',  ( 4.355403765523470305, 8.442910196168369907, 5.601137918078562983 ) ) ;
#4305=CARTESIAN_POINT ( 'NONE',  ( 9.865911304835474738, 1.562606840307950051, 16.04999999999995808 ) ) ;
#4318=CARTESIAN_POINT ( 'NONE',  ( -1.486127417882243895, 9.383039235653816590, 0.2999999999999669598 ) ) ;
#4319=CARTESIAN_POINT ( 'NONE',  ( -4.270415729527831772, -8.486213763410670907, 6.098862081921437195 ) ) ;
#4332=CARTESIAN_POINT ( 'NONE',  ( 10.37072757624895836, -1.642561882922355831, 19.19999999999999574 ) ) ;
#4339=CARTESIAN_POINT ( 'NONE',  ( 9.390499931835536884, -1.439022436064273158, 5.198862081921453715 ) ) ;
#4341=CARTESIAN_POINT ( 'NONE',  ( 10.37072757624895836, -1.642561882922355609, 7.199999999999984190 ) ) ;
#4342=CARTESIAN_POINT ( 'NONE',  ( -9.377220287598998283, -4.724406229267462898, 1.401137918078568134 ) ) ;
#4347=CARTESIAN_POINT ( 'NONE',  ( -7.806708723663830618, -7.806708723663906113, 8.250000000000028422 ) ) ;
#4354=CARTESIAN_POINT ( 'NONE',  ( -6.683790977649319842, 6.751237864895101026, 8.001137918078546463 ) ) ;
#4355=CARTESIAN_POINT ( 'NONE',  ( 8.486213763410640709, 4.270415729527937465, -0.09886208192143307316 ) ) ;
#4368=CARTESIAN_POINT ( 'NONE',  ( 8.922933199037192509, -4.490180821391404287, 20.34886208192140700 ) ) ;
#4369=CARTESIAN_POINT ( 'NONE',  ( -4.579542530753125895, 8.877401133907090625, 10.14886208192142725 ) ) ;
#4370=CARTESIAN_POINT ( 'NONE',  ( -9.355568503977838901, -4.766900247265280832, 14.39999999999996838 ) ) ;
#4384=CARTESIAN_POINT ( 'NONE',  ( 1.642561882922480621, -10.37072757624892638, 13.80000000000003446 ) ) ;
#4393=CARTESIAN_POINT ( 'NONE',  ( 1.513077731352925115, 9.873755945037103743, 1.448862081921441947 ) ) ;
#4395=CARTESIAN_POINT ( 'NONE',  ( 1.642561882922480621, -10.37072757624892638, 4.800000000000026468 ) ) ;
#4396=CARTESIAN_POINT ( 'NONE',  ( -1.595456901104623348, 10.37818827243066622, 2.301137918078551614 ) ) ;
#4400=CARTESIAN_POINT ( 'NONE',  ( -4.766900247265192014, -9.355568503977867323, 8.099999999999996092 ) ) ;
#4407=CARTESIAN_POINT ( 'NONE',  ( -9.375578539472099848, 1.533232399700010351, 16.70113791807854398 ) ) ;
#4408=CARTESIAN_POINT ( 'NONE',  ( -1.486127417882243895, 9.383039235653816590, 18.29999999999998295 ) ) ;
#4421=CARTESIAN_POINT ( 'NONE',  ( -8.900167166472156666, 4.534861676072231340, 2.849999999999968114 ) ) ;
#4422=CARTESIAN_POINT ( 'NONE',  ( -1.513077731352923339, -9.873755945037078874, 11.94886208192145993 ) ) ;
#4424=CARTESIAN_POINT ( 'NONE',  ( 9.837026868206066865, -5.012215536711395636, 16.35000000000000497 ) ) ;
#4433=CARTESIAN_POINT ( 'NONE',  ( 7.424621202458790314, -7.424621202458697944, 10.50000000000000888 ) ) ;
#4436=PRODUCT_DEFINITION_FORMATION_WITH_SPECIFIED_SOURCE ( 'ANY', '', #9805, .NOT_KNOWN. ) ;
#4439=CARTESIAN_POINT ( 'NONE',  ( -10.90442828429183919, -1.727091770866654663, 17.55000000000002913 ) ) ;
#4445=CARTESIAN_POINT ( 'NONE',  ( -1.533232399700100057, 9.375578539472089190, 4.298862081921427603 ) ) ;
#4447=CARTESIAN_POINT ( 'NONE',  ( -9.837026868206066865, 5.012215536711413399, 8.850000000000008527 ) ) ;
#4448=CARTESIAN_POINT ( 'NONE',  ( 9.814260835641038128, -5.056896391392198709, 9.351137918078563871 ) ) ;
#4451=CARTESIAN_POINT ( 'NONE',  ( -1.727091770866549414, -10.90442828429184630, 13.95000000000002593 ) ) ;
#4456=CARTESIAN_POINT ( 'NONE',  ( -4.490180821391513533, 8.922933199037158758, 11.15113791807855215 ) ) ;
#4457=CARTESIAN_POINT ( 'NONE',  ( 8.877401133907127928, -4.579542530753020202, 6.351137918078572753 ) ) ;
#4471=CARTESIAN_POINT ( 'NONE',  ( -5.012215536711506658, 9.837026868206027785, 0.1499999999999952482 ) ) ;
#4472=CARTESIAN_POINT ( 'NONE',  ( 1.562606840307832368, 9.865911304835510265, 9.449999999999988631 ) ) ;
#4473=CARTESIAN_POINT ( 'NONE',  ( 6.751237864895159646, -6.683790977649233689, 8.498862081921462419 ) ) ;
#4474=CARTESIAN_POINT ( 'NONE',  ( -4.766900247265192014, -9.355568503977876205, 14.10000000000000142 ) ) ;
#4484=CARTESIAN_POINT ( 'NONE',  ( 10.90442828429183919, 1.727091770866679532, 19.04999999999997939 ) ) ;
#4489=CARTESIAN_POINT ( 'NONE',  ( 4.766900247265192903, 9.355568503977902850, 18.60000000000000497 ) ) ;
#4503=CARTESIAN_POINT ( 'NONE',  ( 10.89658364409024749, 1.776620879821585897, 17.04886208192142760 ) ) ;
#4505=CARTESIAN_POINT ( 'NONE',  ( 9.837026868206066865, -5.012215536711391195, 10.35000000000002274 ) ) ;
#4506=CARTESIAN_POINT ( 'NONE',  ( 7.842167650704563897, 7.771249796623195039, 14.75113791807856956 ) ) ;
#4510=CARTESIAN_POINT ( 'NONE',  ( -4.766900247265192014, -9.355568503977876205, 14.10000000000000142 ) ) ;
#4512=CARTESIAN_POINT ( 'NONE',  ( -10.90442828429184274, -1.727091770866655773, 8.549999999999963407 ) ) ;
#4515=CARTESIAN_POINT ( 'NONE',  ( -6.683790977649319842, 6.751237864895101026, 17.00113791807859442 ) ) ;
#4516=CARTESIAN_POINT ( 'NONE',  ( -1.612135949262737844, -9.858066664633893694, 3.951137918078560851 ) ) ;
#4527=CARTESIAN_POINT ( 'NONE',  ( 7.424621202458790314, -7.424621202458697944, 1.500000000000001332 ) ) ;
#4528=CARTESIAN_POINT ( 'NONE',  ( -1.486127417882243895, 9.383039235653825472, 9.299999999999975842 ) ) ;
#4529=CARTESIAN_POINT ( 'NONE',  ( -7.027753727702738651, -7.098671581784262941, 15.24886208192144110 ) ) ;
#4540=CARTESIAN_POINT ( 'NONE',  ( -7.424621202458789426, 7.424621202458723701, 15.00000000000001421 ) ) ;
#4545=CARTESIAN_POINT ( 'NONE',  ( 5.012215536711511987, -9.837026868205999364, 13.65000000000003233 ) ) ;
#4557=CARTESIAN_POINT ( 'NONE',  ( 8.442910196168311288, 4.355403765523576887, 7.898862081921404155 ) ) ;
#4559=CARTESIAN_POINT ( 'NONE',  ( -9.837026868206066865, 5.012215536711416064, 5.849999999999989875 ) ) ;
#4560=CARTESIAN_POINT ( 'NONE',  ( 1.595456901104624459, -10.37818827243064668, 9.801137918078557831 ) ) ;
#4564=CARTESIAN_POINT ( 'NONE',  ( -7.424621202458789426, 7.424621202458720148, 3.000000000000002665 ) ) ;
#4568=CARTESIAN_POINT ( 'NONE',  ( 1.439022436064387511, -9.390499931835517344, 12.80113791807860224 ) ) ;
#4569=CARTESIAN_POINT ( 'NONE',  ( 8.877401133907127928, -4.579542530753017537, 9.351137918078563871 ) ) ;
#4579=CARTESIAN_POINT ( 'NONE',  ( -1.486127417882243895, 9.383039235653816590, 3.299999999999969624 ) ) ;
#4580=CARTESIAN_POINT ( 'NONE',  ( -8.922933199037192509, 4.490180821391425603, 15.84886208192146739 ) ) ;
#4590=CARTESIAN_POINT ( 'NONE',  ( -4.766900247265192014, -9.355568503977867323, 11.09999999999999787 ) ) ;
#4593=CARTESIAN_POINT ( 'NONE',  ( -9.859792900771106261, 4.967534682030611215, 12.84886208192143009 ) ) ;
#4597=CARTESIAN_POINT ( 'NONE',  ( -1.562606840307830591, -9.865911304835481843, 10.95000000000000284 ) ) ;
#4605=CARTESIAN_POINT ( 'NONE',  ( -1.513077731352923339, -9.873755945037078874, 8.948862081921467038 ) ) ;
#4608=CARTESIAN_POINT ( 'NONE',  ( 7.842167650704563897, 7.771249796623202144, 11.75113791807857666 ) ) ;
#4615=CARTESIAN_POINT ( 'NONE',  ( -10.36326688006724162, 1.689666864740235308, 7.701137918078540423 ) ) ;
#4616=CARTESIAN_POINT ( 'NONE',  ( 6.683790977649321619, -6.751237864895077045, 0.5011379180785839882 ) ) ;
#4628=CARTESIAN_POINT ( 'NONE',  ( -4.534861676072319270, 8.900167166472117586, 6.149999999999980815 ) ) ;
#4629=CARTESIAN_POINT ( 'NONE',  ( 8.922933199037192509, -4.490180821391404287, 20.34886208192140700 ) ) ;
#4638=CARTESIAN_POINT ( 'NONE',  ( 9.355568503977840678, 4.766900247265305701, 15.90000000000002522 ) ) ;
#4644=CARTESIAN_POINT ( 'NONE',  ( 4.724406229267374968, 9.377220287599064008, 7.598862081921438971 ) ) ;
#4649=CARTESIAN_POINT ( 'NONE',  ( -8.464561979789474222, -4.312909747525728754, 5.400000000000016342 ) ) ;
#4658=CARTESIAN_POINT ( 'NONE',  ( -4.967534682030703586, 9.859792900771061852, 17.15113791807853616 ) ) ;
#4663=CARTESIAN_POINT ( 'NONE',  ( 1.642561882922480621, -10.37072757624891750, 7.800000000000029132 ) ) ;
#4666=CARTESIAN_POINT ( 'NONE',  ( 1.595456901104624459, -10.37818827243064668, 9.801137918078557831 ) ) ;
#4667=CARTESIAN_POINT ( 'NONE',  ( -4.355403765523468529, -8.442910196168346815, 1.101137918078559208 ) ) ;
#4679=APPLICATION_CONTEXT ( 'automotive_design' ) ;
#4680=CARTESIAN_POINT ( 'NONE',  ( 4.534861676072320158, -8.900167166472098046, 13.65000000000003233 ) ) ;
#4681=CARTESIAN_POINT ( 'NONE',  ( -1.513077731352923339, -9.873755945037078874, 17.94886208192144395 ) ) ;
#4683=CARTESIAN_POINT ( 'NONE',  ( -8.900167166472160218, 4.534861676072232228, 2.849999999999968114 ) ) ;
#4693=CARTESIAN_POINT ( 'NONE',  ( -4.724406229267374968, -9.377220287599040915, 9.098862081921437195 ) ) ;
#4698=CARTESIAN_POINT ( 'NONE',  ( 8.900167166472158442, -4.534861676072210912, 7.350000000000000533 ) ) ;
#4699=CARTESIAN_POINT ( 'NONE',  ( -10.37072757624895836, 1.642561882922380923, 17.69999999999999218 ) ) ;
#4706=CARTESIAN_POINT ( 'NONE',  ( 9.837026868206066865, -5.012215536711392083, 1.350000000000015188 ) ) ;
#4707=CARTESIAN_POINT ( 'NONE',  ( -1.727091770866549414, -10.90442828429184630, 1.949999999999996181 ) ) ;
#4713=CARTESIAN_POINT ( 'NONE',  ( -1.727091770866549414, -10.90442828429185695, 4.950000000000017941 ) ) ;
#4717=CARTESIAN_POINT ( 'NONE',  ( -4.809394265263009061, -9.333916720356723928, 4.101137918078561206 ) ) ;
#4718=CARTESIAN_POINT ( 'NONE',  ( 6.683790977649321619, -6.751237864895076157, 18.50113791807859087 ) ) ;
#4729=CARTESIAN_POINT ( 'NONE',  ( -1.486127417882243895, 9.383039235653816590, 12.29999999999997762 ) ) ;
#4730=CARTESIAN_POINT ( 'NONE',  ( 1.513077731352925115, 9.873755945037100190, 13.44886208192141197 ) ) ;
#4733=CARTESIAN_POINT ( 'NONE',  ( -7.063212654743467489, -7.063212654743535879, 2.249999999999986677 ) ) ;
#4743=CARTESIAN_POINT ( 'NONE',  ( -10.37818827243067688, 1.595456901104524761, 6.698862081921455491 ) ) ;
#4749=CARTESIAN_POINT ( 'NONE',  ( -8.464561979789474222, -4.312909747525729642, 14.39999999999996838 ) ) ;
#4750=CARTESIAN_POINT ( 'NONE',  ( 5.012215536711511987, -9.837026868205999364, 16.64999999999999858 ) ) ;
#4756=STYLED_ITEM ( 'NONE', ( #9573 ), #9458 ) ;
#4760=CARTESIAN_POINT ( 'NONE',  ( -9.837026868206066865, 5.012215536711416064, 5.849999999999989875 ) ) ;
#4763=CARTESIAN_POINT ( 'NONE',  ( -9.837026868206070418, 5.012215536711412511, 14.84999999999999609 ) ) ;
#4766=CARTESIAN_POINT ( 'NONE',  ( -7.842167650704559456, -7.771249796623176387, 7.251137918078588207 ) ) ;
#4767=CARTESIAN_POINT ( 'NONE',  ( -4.355403765523468529, -8.442910196168346815, 10.10113791807856742 ) ) ;
#4776=CARTESIAN_POINT ( 'NONE',  ( -4.534861676072319270, 8.900167166472117586, 18.15000000000000924 ) ) ;
#4777=CARTESIAN_POINT ( 'NONE',  ( -1.486127417882243895, 9.383039235653825472, 9.299999999999975842 ) ) ;
#4779=CARTESIAN_POINT ( 'NONE',  ( 8.464561979789474222, 4.312909747525755400, 3.899999999999959055 ) ) ;
#4786=CARTESIAN_POINT ( 'NONE',  ( -1.513077731352923339, -9.873755945037078874, 2.948862081921438616 ) ) ;
#4787=CARTESIAN_POINT ( 'NONE',  ( -7.771249796623103556, -7.842167650704634063, 15.24886208192144110 ) ) ;
#4792=AXIS2_PLACEMENT_3D ( 'NONE', #7204, #9595, #2601 ) ;
#4796=CARTESIAN_POINT ( 'NONE',  ( 9.865911304835478290, 1.562606840307950273, 10.05000000000003268 ) ) ;
#4797=CARTESIAN_POINT ( 'NONE',  ( -10.37072757624895836, 1.642561882922380034, 14.69999999999999041 ) ) ;
#4807=CARTESIAN_POINT ( 'NONE',  ( 7.424621202458790314, -7.424621202458697944, 4.500000000000003553 ) ) ;
#4813=CARTESIAN_POINT ( 'NONE',  ( 1.727091770866551412, 10.90442828429187117, 9.449999999999992184 ) ) ;
#4817=CARTESIAN_POINT ( 'NONE',  ( -1.776620879821455556, -10.89658364409025992, 3.951137918078560851 ) ) ;
#4818=CARTESIAN_POINT ( 'NONE',  ( -1.612135949262737844, -9.858066664633888365, 15.95113791807857595 ) ) ;
#4827=CARTESIAN_POINT ( 'NONE',  ( 1.486127417882244783, -9.383039235653791721, 13.80000000000003446 ) ) ;
#4828=CARTESIAN_POINT ( 'NONE',  ( 8.464561979789474222, 4.312909747525755400, 9.900000000000019895 ) ) ;
#4831=CARTESIAN_POINT ( 'NONE',  ( 1.486127417882244783, -9.383039235653791721, 4.800000000000026468 ) ) ;
#4840=CARTESIAN_POINT ( 'NONE',  ( -6.751237864895158758, 6.683790977649261222, 6.998862081921422451 ) ) ;
#4841=CARTESIAN_POINT ( 'NONE',  ( -10.37818827243067688, 1.595456901104524761, 15.69886208192145816 ) ) ;
#4848=CARTESIAN_POINT ( 'NONE',  ( -1.486127417882243895, 9.383039235653816590, 18.29999999999998295 ) ) ;
#4849=CARTESIAN_POINT ( 'NONE',  ( 9.333916720356675967, 4.809394265263123636, 10.89886208192140771 ) ) ;
#4858=CARTESIAN_POINT ( 'NONE',  ( 9.355568503977840678, 4.766900247265305701, 3.899999999999959055 ) ) ;
#4859=CARTESIAN_POINT ( 'NONE',  ( 9.837026868206066865, -5.012215536711392083, 7.350000000000000533 ) ) ;
#4864=CARTESIAN_POINT ( 'NONE',  ( -10.90442828429184274, -1.727091770866655107, 17.55000000000002913 ) ) ;
#4869=CARTESIAN_POINT ( 'NONE',  ( -10.36326688006724162, 1.689666864740236862, 10.70113791807854220 ) ) ;
#4870=CARTESIAN_POINT ( 'NONE',  ( 1.612135949262739398, 9.858066664633913234, 17.45113791807857240 ) ) ;
#4881=CARTESIAN_POINT ( 'NONE',  ( -6.683790977649319842, 6.751237864895101026, -0.9988620819214586444 ) ) ;
#4882=CARTESIAN_POINT ( 'NONE',  ( -8.464561979789474222, -4.312909747525728754, 5.400000000000016342 ) ) ;
#4885=CARTESIAN_POINT ( 'NONE',  ( 8.464561979789474222, 4.312909747525755400, 0.9000000000000119016 ) ) ;
#4892=CARTESIAN_POINT ( 'NONE',  ( -6.751237864895158758, 6.683790977649260334, 9.998862081921425116 ) ) ;
#4893=CARTESIAN_POINT ( 'NONE',  ( -9.333916720356675967, -4.809394265263096990, 18.39886208192140771 ) ) ;
#4900=CARTESIAN_POINT ( 'NONE',  ( 10.89658364409024749, 1.776620879821585897, 8.048862081921450695 ) ) ;
#4908=CARTESIAN_POINT ( 'NONE',  ( -1.727091770866549414, -10.90442828429184274, 7.950000000000040146 ) ) ;
#4909=CARTESIAN_POINT ( 'NONE',  ( 10.90442828429183919, 1.727091770866678422, 4.049999999999988276 ) ) ;
#4914=CARTESIAN_POINT ( 'NONE',  ( 4.766900247265192903, 9.355568503977911732, 9.599999999999997868 ) ) ;
#4920=CARTESIAN_POINT ( 'NONE',  ( 4.809394265263009061, 9.333916720356739916, 17.60113791807856742 ) ) ;
#4921=CARTESIAN_POINT ( 'NONE',  ( 4.355403765523470305, 8.442910196168369907, 17.60113791807856742 ) ) ;
#4930=CARTESIAN_POINT ( 'NONE',  ( -1.612135949262737844, -9.858066664633893694, 3.951137918078560851 ) ) ;
#4931=CARTESIAN_POINT ( 'NONE',  ( 4.534861676072320158, -8.900167166472098046, 1.650000000000006128 ) ) ;
#4941=CARTESIAN_POINT ( 'NONE',  ( 9.383039235653818366, -1.486127417882130208, 1.200000000000034373 ) ) ;
#4942=CARTESIAN_POINT ( 'NONE',  ( 9.859792900771104485, -4.967534682030585458, 14.34886208192142831 ) ) ;
#4943=UNCERTAINTY_MEASURE_WITH_UNIT (LENGTH_MEASURE( 1.000000000000000082E-05 ), #9420, 'distance_accuracy_value', 'NONE');
#4951=CARTESIAN_POINT ( 'NONE',  ( -7.458344646081709328, 7.390897758835799358, 3.998862081921419342 ) ) ;
#4959=CARTESIAN_POINT ( 'NONE',  ( 5.012215536711511987, -9.837026868205999364, 4.650000000000026112 ) ) ;
#4960=CARTESIAN_POINT ( 'NONE',  ( 1.642561882922480621, -10.37072757624892638, 13.80000000000003446 ) ) ;
#4967=CARTESIAN_POINT ( 'NONE',  ( 1.642561882922480621, -10.37072757624891750, 10.80000000000003268 ) ) ;
#4971=CARTESIAN_POINT ( 'NONE',  ( 1.776620879821457333, 10.89658364409028124, 17.45113791807857240 ) ) ;
#4972=CARTESIAN_POINT ( 'NONE',  ( 9.377220287599001836, 4.724406229267489543, 8.901137918078571687 ) ) ;
#4982=CARTESIAN_POINT ( 'NONE',  ( -1.612135949262737844, -9.858066664633888365, 9.951137918078590161 ) ) ;
#4983=CARTESIAN_POINT ( 'NONE',  ( -7.063212654743466601, -7.063212654743531438, 14.25000000000001243 ) ) ;
#4994=CARTESIAN_POINT ( 'NONE',  ( -4.534861676072319270, 8.900167166472121139, 0.1499999999999952482 ) ) ;
#4995=CARTESIAN_POINT ( 'NONE',  ( 10.89658364409024749, 1.776620879821585897, 17.04886208192142760 ) ) ;
#5001=CARTESIAN_POINT ( 'NONE',  ( -4.534861676072319270, 8.900167166472122915, 15.14999999999998614 ) ) ;
#5002=CARTESIAN_POINT ( 'NONE',  ( 7.771249796623105333, 7.842167650704653603, 4.748862081921425116 ) ) ;
#5009=CARTESIAN_POINT ( 'NONE',  ( 1.727091770866550968, 10.90442828429186761, 6.449999999999969091 ) ) ;
#5016=CARTESIAN_POINT ( 'NONE',  ( -4.967534682030703586, 9.859792900771058299, 14.15113791807854327 ) ) ;
#5017=CARTESIAN_POINT ( 'NONE',  ( -10.36326688006724162, 1.689666864740236640, 4.701137918078535982 ) ) ;
#5023=CARTESIAN_POINT ( 'NONE',  ( 10.37072757624895836, -1.642561882922355609, 7.199999999999984190 ) ) ;
#5031=CARTESIAN_POINT ( 'NONE',  ( -1.439022436064386845, 9.390499931835535108, 5.301137918078554279 ) ) ;
#5032=CARTESIAN_POINT ( 'NONE',  ( 6.717514421272239744, -6.717514421272154479, 19.50000000000001776 ) ) ;
#5043=CARTESIAN_POINT ( 'NONE',  ( 7.027753727702739539, 7.098671581784288698, 19.74886208192143044 ) ) ;
#5044=CARTESIAN_POINT ( 'NONE',  ( -4.579542530753125895, 8.877401133907090625, 7.148862081921437017 ) ) ;
#5051=CARTESIAN_POINT ( 'NONE',  ( -1.689666864740335228, 10.36326688006722740, 4.298862081921427603 ) ) ;
#5052=EDGE_LOOP ( 'NONE', ( #774, #1329, #9468, #3141 ) ) ;
#5057=CARTESIAN_POINT ( 'NONE',  ( -7.424621202458789426, 7.424621202458724589, 6.000000000000005329 ) ) ;
#5064=CARTESIAN_POINT ( 'NONE',  ( 1.595456901104624459, -10.37818827243065201, 12.80113791807860224 ) ) ;
#5065=CARTESIAN_POINT ( 'NONE',  ( -4.967534682030703586, 9.859792900771061852, 2.151137918078574796 ) ) ;
#5069=CARTESIAN_POINT ( 'NONE',  ( 10.37072757624895836, -1.642561882922355609, 10.19999999999998685 ) ) ;
#5076=CARTESIAN_POINT ( 'NONE',  ( -4.490180821391513533, 8.922933199037158758, 2.151137918078574796 ) ) ;
#5077=CARTESIAN_POINT ( 'NONE',  ( 9.865911304835474738, 1.562606840307950051, 13.04999999999999538 ) ) ;
#5086=( LENGTH_UNIT ( ) NAMED_UNIT ( * ) SI_UNIT ( .MILLI., .METRE. ) );
#5090=CARTESIAN_POINT ( 'NONE',  ( -6.717514421272238856, 6.717514421272181124, 0.000000000000000000 ) ) ;
#5091=CARTESIAN_POINT ( 'NONE',  ( 8.442910196168311288, 4.355403765523574222, 10.89886208192140771 ) ) ;
#5104=CARTESIAN_POINT ( 'NONE',  ( -10.37072757624895836, 1.642561882922380034, 14.69999999999999041 ) ) ;
#5112=CARTESIAN_POINT ( 'NONE',  ( -1.689666864740335228, 10.36326688006723451, 16.29886208192143471 ) ) ;
#5114=CARTESIAN_POINT ( 'NONE',  ( 4.766900247265192903, 9.355568503977902850, 3.599999999999992095 ) ) ;
#5115=CARTESIAN_POINT ( 'NONE',  ( -7.842167650704559456, -7.771249796623180828, 4.251137918078595312 ) ) ;
#5123=CARTESIAN_POINT ( 'NONE',  ( -5.012215536711506658, 9.837026868206027785, 3.149999999999957723 ) ) ;
#5134=CARTESIAN_POINT ( 'NONE',  ( 7.098671581784200768, 7.027753727702831021, 2.751137918078555789 ) ) ;
#5135=CARTESIAN_POINT ( 'NONE',  ( -7.063212654743466601, -7.063212654743531438, 17.25000000000003553 ) ) ;
#5145=CARTESIAN_POINT ( 'NONE',  ( -9.390499931835536884, 1.439022436064298249, 18.69886208192145816 ) ) ;
#5146=CARTESIAN_POINT ( 'NONE',  ( 4.579542530753127672, -8.877401133907065756, 5.648862081921440570 ) ) ;
#5148=CARTESIAN_POINT ( 'NONE',  ( 1.727091770866550968, 10.90442828429187294, 12.44999999999995666 ) ) ;
#5157=ORIENTED_EDGE ( 'NONE', *, *, #8032, .F. ) ;
#5162=CARTESIAN_POINT ( 'NONE',  ( -1.689666864740335228, 10.36326688006723273, 1.298862081921425604 ) ) ;
#5168=CARTESIAN_POINT ( 'NONE',  ( 9.837026868206070418, -5.012215536711392083, 19.34999999999997300 ) ) ;
#5171=CARTESIAN_POINT ( 'NONE',  ( 4.579542530753127672, -8.877401133907065756, 2.648862081921448119 ) ) ;
#5173=CARTESIAN_POINT ( 'NONE',  ( -10.37072757624895836, 1.642561882922380923, 2.699999999999980194 ) ) ;
#5174=CARTESIAN_POINT ( 'NONE',  ( 4.809394265263009061, 9.333916720356734587, 2.601137918078560762 ) ) ;
#5178=CARTESIAN_POINT ( 'NONE',  ( 9.355568503977840678, 4.766900247265305701, 6.899999999999961275 ) ) ;
#5183=CARTESIAN_POINT ( 'NONE',  ( 8.486213763410640709, 4.270415729527937465, 14.90113791807857879 ) ) ;
#5184=CARTESIAN_POINT ( 'NONE',  ( 6.717514421272239744, -6.717514421272154479, 13.50000000000001243 ) ) ;
#5196=CARTESIAN_POINT ( 'NONE',  ( -1.486127417882243895, 9.383039235653825472, 6.299999999999972289 ) ) ;
#5197=CARTESIAN_POINT ( 'NONE',  ( -4.579542530753125895, 8.877401133907083519, 4.148862081921444123 ) ) ;
#5198=CARTESIAN_POINT ( 'NONE',  ( -9.837026868206066865, 5.012215536711413399, 14.84999999999999787 ) ) ;
#5206=CARTESIAN_POINT ( 'NONE',  ( -9.837026868206066865, 5.012215536711416064, 17.85000000000001918 ) ) ;
#5210=CARTESIAN_POINT ( 'NONE',  ( -4.766900247265192014, -9.355568503977876205, 17.10000000000000497 ) ) ;
#5217=CARTESIAN_POINT ( 'NONE',  ( -9.859792900771106261, 4.967534682030611215, 18.84886208192146029 ) ) ;
#5218=CARTESIAN_POINT ( 'NONE',  ( -9.355568503977838901, -4.766900247265279944, 5.400000000000016342 ) ) ;
#5219=CARTESIAN_POINT ( 'NONE',  ( 1.776620879821457333, 10.89658364409028124, 11.45113791807854220 ) ) ;
#5222=CARTESIAN_POINT ( 'NONE',  ( 10.37072757624895836, -1.642561882922355609, 4.199999999999981526 ) ) ;
#5227=CARTESIAN_POINT ( 'NONE',  ( 7.098671581784200768, 7.027753727702831021, 17.75113791807856245 ) ) ;
#5228=CARTESIAN_POINT ( 'NONE',  ( 4.355403765523470305, 8.442910196168364578, 2.601137918078560762 ) ) ;
#5239=CARTESIAN_POINT ( 'NONE',  ( -9.383039235653820143, 1.486127417882155521, 8.700000000000041922 ) ) ;
#5240=CARTESIAN_POINT ( 'NONE',  ( -9.858066664633883036, -1.612135949262833101, 12.54886208192144004 ) ) ;
#5241=CARTESIAN_POINT ( 'NONE',  ( -9.355568503977838901, -4.766900247265279944, 11.39999999999996660 ) ) ;
#5248=CARTESIAN_POINT ( 'NONE',  ( 1.727091770866550968, 10.90442828429187294, 12.44999999999995666 ) ) ;
#5252=CARTESIAN_POINT ( 'NONE',  ( 7.424621202458790314, -7.424621202458697944, 13.50000000000001243 ) ) ;
#5261=CARTESIAN_POINT ( 'NONE',  ( -10.89658364409024749, -1.776620879821559917, 18.54886208192142405 ) ) ;
#5262=CARTESIAN_POINT ( 'NONE',  ( 10.90442828429183919, 1.727091770866679532, 10.05000000000002736 ) ) ;
#5263=CARTESIAN_POINT ( 'NONE',  ( -10.36326688006724162, 1.689666864740235308, 16.70113791807854398 ) ) ;
#5267=( BOUNDED_SURFACE ( )  B_SPLINE_SURFACE ( 3, 2, ( 
 ( #828, #3832, #5478, #3048, #734, #7903, #2376, #5527, #6190, #4706, #8686, #1608, #7133, #9365, #3207, #6341, #2277, #5424, #8736, #1656, #8581, #779, #3882, #9521, #5573, #7381, #4858, #3448, #8847, #1804, #1135, #4959, #1908, #2624, #8111, #8054, #2581, #4230, #209, #4184, #5057, #2529, #5770, #5009, #5724, #1858, #1757, #8155, #1089, #5678, #7285, #7334, #307, #4908, #150, #6590, #984, #4133, #6541, #5822, #1040, #6494, #3359, #9672, #8892, #9773, #2676, #258, #3405, #8999, #8203, #4280, #5627, #9720, #8945, #7432, #3252, #6392, #9570, #2473, #8793, #1713, #8005, #935, #6446, #4080, #7230, #3305, #9626, #9867, #5252, #4545, #4384, #2166, #9095, #9199, #1281, #510, #5104, #5972, #9970, #2878, #7585, #9246, #8408, #3656, #6683, #9822, #2928, #8313, #361, #3508, #6845, #1233, #5210, #8256, #6638, #4439, #411, #2724, #6793, #7643, #563, #7535, #4489, #3711, #1183, #5310, #4332, #1335, #7483 ),
 ( #6020, #462, #5162, #10016, #2008, #5919, #2109, #6071, #8467, #3555, #1392, #5867, #8360, #3601, #6733, #9924, #2827, #9045, #1955, #9150, #2772, #2057, #3191, #5514, #10065, #6175, #5463, #9402, #8567, #2414, #5560, #7799, #1593, #3866, #8674, #617, #667, #814, #4743, #2313, #1490, #6955, #2361, #1643, #4644, #9508, #9351, #6276, #8624, #7839, #2216, #3083, #7058, #10220, #4693, #6327, #7889, #766, #3820, #6898, #34, #5409, #7698, #3764, #3967, #720, #1545, #5362, #2982, #3912, #7747, #6128, #3131, #7118, #8721, #7009, #9302, #8518, #1442, #4593, #10119, #3034, #2261, #6226, #10167, #9459, #6377, #9556, #7166, #4022, #2461, #84, #3239, #5609, #8779, #4787, #870, #7942, #1289, #6857, #2939, #6740, #5112, #4287, #2887, #8421, #5876, #4503, #9876, #2836, #2181, #5980, #6082, #3668, #9159, #9106, #3610, #5261, #1239, #5217, #9259, #3561, #6803, #6029, #9932, #9209, #2780, #2120, #1348, #6692, #8321 ),
 ( #7656, #575, #3720, #4393, #9054, #10029, #5324, #6645, #5928, #2066, #8369, #5171, #8479, #7441, #7543, #367, #469, #3517, #9830, #7492, #2730, #1963, #4445, #7596, #2015, #8266, #1189, #521, #4339, #9980, #418, #2459, #1696, #6138, #7023, #918, #134, #8774, #190, #6427, #4840, #681, #629, #4117, #9363, #1404, #4557, #8039, #2275, #6237, #9314, #7708, #5607, #4605, #3777, #7991, #8830, #1741, #8579, #5662, #4892, #2227, #6477, #5373, #9609, #8529, #10181, #2513, #968, #3285, #7263, #5422, #6187, #3343, #10130, #6968, #6909, #10079, #2995, #3830, #3046, #732, #3880, #3097, #9414, #9702, #8875, #7468, #2756, #240, #9079, #4214, #7414, #6719, #342, #7520, #8238, #3492, #3435, #8188, #9852, #5807, #9807, #444, #8138, #1166, #396, #1120, #3542, #7366, #6668, #5904, #1074, #2660, #2709, #1990, #292, #5754, #5145, #6572, #9755, #1940, #1217, #6622, #1894, #5043, #4266, #5852, #8296, #4368, #9029 ),
 ( #5090, #4994, #4318, #3585, #9903, #2810, #1790, #4169, #4941, #8090, #1019, #2609, #7317, #3390, #6524, #8923, #1840, #5293, #6773, #4421, #7571, #8450, #4579, #1377, #9340, #6996, #9290, #2911, #10109, #3803, #547, #10156, #6055, #8503, #5956, #6164, #9958, #492, #3021, #2090, #9230, #4628, #5196, #2861, #9185, #2039, #9136, #8344, #7786, #8393, #708, #5396, #3638, #1318, #6007, #2249, #6939, #2146, #5239, #8554, #1480, #3855, #4528, #4472, #7685, #7628, #7736, #654, #3695, #1263, #6829, #10003, #601, #3747, #6883, #10052, #2964, #6112, #2203, #5351, #1429, #1531, #4729, #4106, #7875, #802, #3950, #6213, #855, #5447, #1684, #4680, #4827, #2448, #23, #7980, #7096, #9593, #1732, #8025, #6260, #4055, #5548, #1629, #5501, #8818, #6313, #7828, #8707, #2500, #2351, #4007, #3273, #7154, #9494, #6414, #7925, #5594, #7202, #7047, #3177, #4776, #907, #121, #10206, #1581, #2399, #72, #3226, #6363, #5649 ),
 ( #4881, #956, #9541, #9445, #8757, #8608, #756, #3903, #7250, #3070, #9389, #2302, #3119, #8660, #8176, #2552, #9019, #1777, #1928, #9796, #7355, #5076, #1062, #6658, #9068, #5134, #3379, #1153, #2648, #8971, #2599, #5889, #3423, #4930, #5796, #9841, #9690, #1110, #381, #4254, #6561, #3533, #5031, #2700, #4304, #4155, #278, #1883, #8226, #7455, #7304, #8911, #8077, #1976, #6609, #6512, #7403, #2744, #8281, #1203, #4354, #5696, #173, #4203, #8864, #226, #5742, #3331, #9646, #327, #1827, #3476, #1007, #4982, #8128, #5841, #6468, #2898, #642, #8543, #588, #4456, #1418, #5337, #2079, #1466, #7613, #10039, #7506, #7722, #8332, #5943, #4568, #3621, #534, #6151, #6706, #1250, #479, #3572, #431, #9890, #9327, #9944, #2237, #6921, #5183, #2849, #7556, #3791, #8492, #3683, #9123, #10096, #3007, #5383, #6818, #2025, #4407, #2793, #4515, #6758, #5994, #9992, #9173, #5227, #6095, #8381, #1304, #6042, #9218 ),
 ( #6869, #2133, #5275, #8438, #1362, #7672, #3733, #2951, #9276, #2190, #6352, #3940, #3216, #3110, #9531, #2436, #7035, #8648, #8696, #5582, #6250, #1519, #8745, #9427, #10195, #7912, #7191, #2387, #7863, #2338, #1571, #790, #1668, #4817, #4717, #5537, #7967, #108, #897, #6981, #5490, #1618, #6301, #7084, #9579, #2484, #6, #4045, #3163, #3261, #7770, #7817, #6403, #5638, #9484, #4766, #3891, #8805, #4615, #839, #697, #3997, #3844, #7142, #60, #9376, #10143, #3057, #6201, #2290, #5433, #8592, #4666, #744, #946, #4288, #9681, #5878, #4869, #8212, #2588, #6549, #9635, #8014, #2633, #1765, #1723, #5781, #9005, #1916, #8900, #5829, #5064, #2539, #6647, #6456, #9785, #5685, #7343, #2686, #1142, #5016, #1868, #5733, #6501, #7443, #216, #7293, #8162, #3457, #370, #3367, #8855, #3519, #1097, #8065, #1814, #9832, #2732, #4092, #7241, #159, #3316, #4971, #4920, #993, #4142, #8120, #1050, #4194, #266 ),
 ( #3413, #316, #9732, #8956, #4238, #7389, #6599, #2941, #6858, #3611, #2997, #9161, #1350, #9056, #9261, #9878, #7494, #6084, #5173, #2068, #7710, #8268, #2782, #2016, #5114, #1964, #1191, #631, #1241, #3779, #8482, #6693, #4395, #9108, #2183, #5326, #5218, #420, #1406, #4559, #6911, #8370, #3563, #523, #5930, #7659, #577, #6742, #4341, #10081, #2838, #3722, #8323, #7544, #470, #7598, #9935, #5982, #1291, #4447, #3671, #6805, #9982, #2888, #6030, #9210, #2122, #5262, #8422, #4505, #4433, #1437, #2213, #10012, #4590, #3707, #9347, #1487, #7796, #6016, #3814, #5305, #1387, #5248, #8562, #6067, #7581, #8462, #2257, #2104, #3760, #3030, #6894, #9241, #6172, #7694, #5359, #6951, #6788, #2923, #4540, #7744, #10116, #9966, #2823, #9146, #4638, #8403, #717, #5405, #504, #1328, #2873, #3864, #7004, #2159, #1275, #5968, #2053, #5206, #613, #3651, #10062, #9195, #663, #8356, #558, #4484, #7639, #6840, #2975 ) ),
 .UNSPECIFIED., .T., .F., .F. ) 
 B_SPLINE_SURFACE_WITH_KNOTS ( ( 4, 3, 4 ),
 ( 3, 2, 2, 2, 2, 2, 2, 2, 2, 2, 2, 2, 2, 2, 2, 2, 2, 2, 2, 2, 2, 2, 2, 2, 2, 2, 2, 2, 2, 2, 2, 2, 2, 2, 2, 2, 2, 2, 2, 2, 2, 2, 2, 2, 2, 2, 2, 2, 2, 2, 2, 2, 2, 2, 2, 2, 2, 2, 2, 2, 2, 2, 2, 2, 2, 3 ),
 ( 0.000000000000000000, 0.5000000000000000000, 1.000000000000000000 ),
 ( 0.000000000000000000, 0.01428571428571428527, 0.02857142857142857054, 0.04285714285714285754, 0.05714285714285714107, 0.07142857142857142461, 0.08571428571428571508, 0.1000000000000000056, 0.1142857142857142821, 0.1285714285714285587, 0.1428571428571428492, 0.1571428571428571397, 0.1714285714285714302, 0.1857142857142857206, 0.2000000000000000111, 0.2142857142857142738, 0.2285714285714285643, 0.2428571428571428548, 0.2571428571428571175, 0.2714285714285714080, 0.2857142857142856984, 0.2999999999999999889, 0.3142857142857142794, 0.3285714285714285698, 0.3428571428571428603, 0.3571428571428571508, 0.3714285714285714413, 0.3857142857142857317, 0.4000000000000000222, 0.4142857142857143127, 0.4285714285714285476, 0.4428571428571428381, 0.4571428571428571286, 0.4714285714285714191, 0.4857142857142857095, 0.5000000000000000000, 0.5142857142857142350, 0.5285714285714285809, 0.5428571428571428159, 0.5571428571428571619, 0.5714285714285713969, 0.5857142857142857428, 0.5999999999999999778, 0.6142857142857143238, 0.6285714285714285587, 0.6428571428571429047, 0.6571428571428571397, 0.6714285714285713746, 0.6857142857142857206, 0.6999999999999999556, 0.7142857142857143016, 0.7285714285714285365, 0.7428571428571428825, 0.7571428571428571175, 0.7714285714285714635, 0.7857142857142856984, 0.8000000000000000444, 0.8142857142857142794, 0.8285714285714286254, 0.8428571428571428603, 0.8571428571428570953, 0.8714285714285714413, 0.8857142857142856762, 0.9000000000000000222, 0.9142857142857142572, 0.9285714285714286031 ),
 .UNSPECIFIED. ) 
 GEOMETRIC_REPRESENTATION_ITEM ( )  RATIONAL_B_SPLINE_SURFACE ( (
 ( 1.000000000000000000, 0.9510565162951535312, 1.000000000000000000, 0.9510565162951535312, 1.000000000000000000, 0.9510565162951535312, 1.000000000000000000, 0.9510565162951535312, 1.000000000000000000, 0.9510565162951535312, 1.000000000000000000, 0.9510565162951535312, 1.000000000000000000, 0.9510565162951535312, 1.000000000000000000, 0.9510565162951535312, 1.000000000000000000, 0.9510565162951535312, 1.000000000000000000, 0.9510565162951535312, 1.000000000000000000, 0.9510565162951535312, 1.000000000000000000, 0.9510565162951535312, 1.000000000000000000, 0.9510565162951535312, 1.000000000000000000, 0.9510565162951535312, 1.000000000000000000, 0.9510565162951535312, 1.000000000000000000, 0.9510565162951535312, 1.000000000000000000, 0.9510565162951535312, 1.000000000000000000, 0.9510565162951535312, 1.000000000000000000, 0.9510565162951535312, 1.000000000000000000, 0.9510565162951535312, 1.000000000000000000, 0.9510565162951535312, 1.000000000000000000, 0.9510565162951535312, 1.000000000000000000, 0.9510565162951535312, 1.000000000000000000, 0.9510565162951535312, 1.000000000000000000, 0.9510565162951535312, 1.000000000000000000, 0.9510565162951535312, 1.000000000000000000, 0.9510565162951535312, 1.000000000000000000, 0.9510565162951535312, 1.000000000000000000, 0.9510565162951535312, 1.000000000000000000, 0.9510565162951535312, 1.000000000000000000, 0.9510565162951535312, 1.000000000000000000, 0.9510565162951535312, 1.000000000000000000, 0.9510565162951535312, 1.000000000000000000, 0.9510565162951535312, 1.000000000000000000, 0.9510565162951535312, 1.000000000000000000, 0.9510565162951535312, 1.000000000000000000, 0.9510565162951535312, 1.000000000000000000, 0.9510565162951535312, 1.000000000000000000, 0.9510565162951535312, 1.000000000000000000, 0.9510565162951535312, 1.000000000000000000, 0.9510565162951535312, 1.000000000000000000, 0.9510565162951535312, 1.000000000000000000, 0.9510565162951535312, 1.000000000000000000, 0.9510565162951535312, 1.000000000000000000, 0.9510565162951535312, 1.000000000000000000, 0.9510565162951535312, 1.000000000000000000, 0.9510565162951535312, 1.000000000000000000, 0.9510565162951535312, 1.000000000000000000, 0.9510565162951535312, 1.000000000000000000, 0.9510565162951535312, 1.000000000000000000, 0.9510565162951535312, 1.000000000000000000, 0.9510565162951535312, 1.000000000000000000, 0.9510565162951535312, 1.000000000000000000, 0.9510565162951535312, 1.000000000000000000, 0.9510565162951535312, 1.000000000000000000, 0.9510565162951535312, 1.000000000000000000, 0.9510565162951535312, 1.000000000000000000, 0.9510565162951535312, 1.000000000000000000, 0.9510565162951535312, 1.000000000000000000, 0.9510565162951535312, 1.000000000000000000, 0.9510565162951535312, 1.000000000000000000, 0.9510565162951535312, 1.000000000000000000, 0.9510565162951535312, 1.000000000000000000, 0.9510565162951535312, 1.000000000000000000, 0.9510565162951535312, 1.000000000000000000),
 ( 0.3333333333333333703, 0.3170188387650512141, 0.3333333333333333703, 0.3170188387650512141, 0.3333333333333333703, 0.3170188387650512141, 0.3333333333333333703, 0.3170188387650512141, 0.3333333333333333703, 0.3170188387650512141, 0.3333333333333333703, 0.3170188387650512141, 0.3333333333333333703, 0.3170188387650512141, 0.3333333333333333703, 0.3170188387650512141, 0.3333333333333333703, 0.3170188387650512141, 0.3333333333333333703, 0.3170188387650512141, 0.3333333333333333703, 0.3170188387650512141, 0.3333333333333333703, 0.3170188387650512141, 0.3333333333333333703, 0.3170188387650512141, 0.3333333333333333703, 0.3170188387650512141, 0.3333333333333333703, 0.3170188387650512141, 0.3333333333333333703, 0.3170188387650512141, 0.3333333333333333703, 0.3170188387650512141, 0.3333333333333333703, 0.3170188387650512141, 0.3333333333333333703, 0.3170188387650512141, 0.3333333333333333703, 0.3170188387650512141, 0.3333333333333333703, 0.3170188387650512141, 0.3333333333333333703, 0.3170188387650512141, 0.3333333333333333703, 0.3170188387650512141, 0.3333333333333333703, 0.3170188387650512141, 0.3333333333333333703, 0.3170188387650512141, 0.3333333333333333703, 0.3170188387650512141, 0.3333333333333333703, 0.3170188387650512141, 0.3333333333333333703, 0.3170188387650512141, 0.3333333333333333703, 0.3170188387650512141, 0.3333333333333333703, 0.3170188387650512141, 0.3333333333333333703, 0.3170188387650512141, 0.3333333333333333703, 0.3170188387650512141, 0.3333333333333333703, 0.3170188387650512141, 0.3333333333333333703, 0.3170188387650512141, 0.3333333333333333703, 0.3170188387650512141, 0.3333333333333333703, 0.3170188387650512141, 0.3333333333333333703, 0.3170188387650512141, 0.3333333333333333703, 0.3170188387650512141, 0.3333333333333333703, 0.3170188387650512141, 0.3333333333333333703, 0.3170188387650512141, 0.3333333333333333703, 0.3170188387650512141, 0.3333333333333333703, 0.3170188387650512141, 0.3333333333333333703, 0.3170188387650512141, 0.3333333333333333703, 0.3170188387650512141, 0.3333333333333333703, 0.3170188387650512141, 0.3333333333333333703, 0.3170188387650512141, 0.3333333333333333703, 0.3170188387650512141, 0.3333333333333333703, 0.3170188387650512141, 0.3333333333333333703, 0.3170188387650512141, 0.3333333333333333703, 0.3170188387650512141, 0.3333333333333333703, 0.3170188387650512141, 0.3333333333333333703, 0.3170188387650512141, 0.3333333333333333703, 0.3170188387650512141, 0.3333333333333333703, 0.3170188387650512141, 0.3333333333333333703, 0.3170188387650512141, 0.3333333333333333703, 0.3170188387650512141, 0.3333333333333333703, 0.3170188387650512141, 0.3333333333333333703, 0.3170188387650512141, 0.3333333333333333703, 0.3170188387650512141, 0.3333333333333333703, 0.3170188387650512141, 0.3333333333333333703, 0.3170188387650512141, 0.3333333333333333703, 0.3170188387650512141, 0.3333333333333333703, 0.3170188387650512141, 0.3333333333333333703, 0.3170188387650512141, 0.3333333333333333703, 0.3170188387650512141, 0.3333333333333333703),
 ( 0.3333333333333333703, 0.3170188387650512141, 0.3333333333333333703, 0.3170188387650512141, 0.3333333333333333703, 0.3170188387650512141, 0.3333333333333333703, 0.3170188387650512141, 0.3333333333333333703, 0.3170188387650512141, 0.3333333333333333703, 0.3170188387650512141, 0.3333333333333333703, 0.3170188387650512141, 0.3333333333333333703, 0.3170188387650512141, 0.3333333333333333703, 0.3170188387650512141, 0.3333333333333333703, 0.3170188387650512141, 0.3333333333333333703, 0.3170188387650512141, 0.3333333333333333703, 0.3170188387650512141, 0.3333333333333333703, 0.3170188387650512141, 0.3333333333333333703, 0.3170188387650512141, 0.3333333333333333703, 0.3170188387650512141, 0.3333333333333333703, 0.3170188387650512141, 0.3333333333333333703, 0.3170188387650512141, 0.3333333333333333703, 0.3170188387650512141, 0.3333333333333333703, 0.3170188387650512141, 0.3333333333333333703, 0.3170188387650512141, 0.3333333333333333703, 0.3170188387650512141, 0.3333333333333333703, 0.3170188387650512141, 0.3333333333333333703, 0.3170188387650512141, 0.3333333333333333703, 0.3170188387650512141, 0.3333333333333333703, 0.3170188387650512141, 0.3333333333333333703, 0.3170188387650512141, 0.3333333333333333703, 0.3170188387650512141, 0.3333333333333333703, 0.3170188387650512141, 0.3333333333333333703, 0.3170188387650512141, 0.3333333333333333703, 0.3170188387650512141, 0.3333333333333333703, 0.3170188387650512141, 0.3333333333333333703, 0.3170188387650512141, 0.3333333333333333703, 0.3170188387650512141, 0.3333333333333333703, 0.3170188387650512141, 0.3333333333333333703, 0.3170188387650512141, 0.3333333333333333703, 0.3170188387650512141, 0.3333333333333333703, 0.3170188387650512141, 0.3333333333333333703, 0.3170188387650512141, 0.3333333333333333703, 0.3170188387650512141, 0.3333333333333333703, 0.3170188387650512141, 0.3333333333333333703, 0.3170188387650512141, 0.3333333333333333703, 0.3170188387650512141, 0.3333333333333333703, 0.3170188387650512141, 0.3333333333333333703, 0.3170188387650512141, 0.3333333333333333703, 0.3170188387650512141, 0.3333333333333333703, 0.3170188387650512141, 0.3333333333333333703, 0.3170188387650512141, 0.3333333333333333703, 0.3170188387650512141, 0.3333333333333333703, 0.3170188387650512141, 0.3333333333333333703, 0.3170188387650512141, 0.3333333333333333703, 0.3170188387650512141, 0.3333333333333333703, 0.3170188387650512141, 0.3333333333333333703, 0.3170188387650512141, 0.3333333333333333703, 0.3170188387650512141, 0.3333333333333333703, 0.3170188387650512141, 0.3333333333333333703, 0.3170188387650512141, 0.3333333333333333703, 0.3170188387650512141, 0.3333333333333333703, 0.3170188387650512141, 0.3333333333333333703, 0.3170188387650512141, 0.3333333333333333703, 0.3170188387650512141, 0.3333333333333333703, 0.3170188387650512141, 0.3333333333333333703, 0.3170188387650512141, 0.3333333333333333703, 0.3170188387650512141, 0.3333333333333333703, 0.3170188387650512141, 0.3333333333333333703, 0.3170188387650512141, 0.3333333333333333703),
 ( 1.000000000000000000, 0.9510565162951535312, 1.000000000000000000, 0.9510565162951535312, 1.000000000000000000, 0.9510565162951535312, 1.000000000000000000, 0.9510565162951535312, 1.000000000000000000, 0.9510565162951535312, 1.000000000000000000, 0.9510565162951535312, 1.000000000000000000, 0.9510565162951535312, 1.000000000000000000, 0.9510565162951535312, 1.000000000000000000, 0.9510565162951535312, 1.000000000000000000, 0.9510565162951535312, 1.000000000000000000, 0.9510565162951535312, 1.000000000000000000, 0.9510565162951535312, 1.000000000000000000, 0.9510565162951535312, 1.000000000000000000, 0.9510565162951535312, 1.000000000000000000, 0.9510565162951535312, 1.000000000000000000, 0.9510565162951535312, 1.000000000000000000, 0.9510565162951535312, 1.000000000000000000, 0.9510565162951535312, 1.000000000000000000, 0.9510565162951535312, 1.000000000000000000, 0.9510565162951535312, 1.000000000000000000, 0.9510565162951535312, 1.000000000000000000, 0.9510565162951535312, 1.000000000000000000, 0.9510565162951535312, 1.000000000000000000, 0.9510565162951535312, 1.000000000000000000, 0.9510565162951535312, 1.000000000000000000, 0.9510565162951535312, 1.000000000000000000, 0.9510565162951535312, 1.000000000000000000, 0.9510565162951535312, 1.000000000000000000, 0.9510565162951535312, 1.000000000000000000, 0.9510565162951535312, 1.000000000000000000, 0.9510565162951535312, 1.000000000000000000, 0.9510565162951535312, 1.000000000000000000, 0.9510565162951535312, 1.000000000000000000, 0.9510565162951535312, 1.000000000000000000, 0.9510565162951535312, 1.000000000000000000, 0.9510565162951535312, 1.000000000000000000, 0.9510565162951535312, 1.000000000000000000, 0.9510565162951535312, 1.000000000000000000, 0.9510565162951535312, 1.000000000000000000, 0.9510565162951535312, 1.000000000000000000, 0.9510565162951535312, 1.000000000000000000, 0.9510565162951535312, 1.000000000000000000, 0.9510565162951535312, 1.000000000000000000, 0.9510565162951535312, 1.000000000000000000, 0.9510565162951535312, 1.000000000000000000, 0.9510565162951535312, 1.000000000000000000, 0.9510565162951535312, 1.000000000000000000, 0.9510565162951535312, 1.000000000000000000, 0.9510565162951535312, 1.000000000000000000, 0.9510565162951535312, 1.000000000000000000, 0.9510565162951535312, 1.000000000000000000, 0.9510565162951535312, 1.000000000000000000, 0.9510565162951535312, 1.000000000000000000, 0.9510565162951535312, 1.000000000000000000, 0.9510565162951535312, 1.000000000000000000, 0.9510565162951535312, 1.000000000000000000, 0.9510565162951535312, 1.000000000000000000, 0.9510565162951535312, 1.000000000000000000, 0.9510565162951535312, 1.000000000000000000, 0.9510565162951535312, 1.000000000000000000, 0.9510565162951535312, 1.000000000000000000, 0.9510565162951535312, 1.000000000000000000, 0.9510565162951535312, 1.000000000000000000, 0.9510565162951535312, 1.000000000000000000, 0.9510565162951535312, 1.000000000000000000),
 ( 0.3333333333333333703, 0.3170188387650512141, 0.3333333333333333703, 0.3170188387650512141, 0.3333333333333333703, 0.3170188387650512141, 0.3333333333333333703, 0.3170188387650512141, 0.3333333333333333703, 0.3170188387650512141, 0.3333333333333333703, 0.3170188387650512141, 0.3333333333333333703, 0.3170188387650512141, 0.3333333333333333703, 0.3170188387650512141, 0.3333333333333333703, 0.3170188387650512141, 0.3333333333333333703, 0.3170188387650512141, 0.3333333333333333703, 0.3170188387650512141, 0.3333333333333333703, 0.3170188387650512141, 0.3333333333333333703, 0.3170188387650512141, 0.3333333333333333703, 0.3170188387650512141, 0.3333333333333333703, 0.3170188387650512141, 0.3333333333333333703, 0.3170188387650512141, 0.3333333333333333703, 0.3170188387650512141, 0.3333333333333333703, 0.3170188387650512141, 0.3333333333333333703, 0.3170188387650512141, 0.3333333333333333703, 0.3170188387650512141, 0.3333333333333333703, 0.3170188387650512141, 0.3333333333333333703, 0.3170188387650512141, 0.3333333333333333703, 0.3170188387650512141, 0.3333333333333333703, 0.3170188387650512141, 0.3333333333333333703, 0.3170188387650512141, 0.3333333333333333703, 0.3170188387650512141, 0.3333333333333333703, 0.3170188387650512141, 0.3333333333333333703, 0.3170188387650512141, 0.3333333333333333703, 0.3170188387650512141, 0.3333333333333333703, 0.3170188387650512141, 0.3333333333333333703, 0.3170188387650512141, 0.3333333333333333703, 0.3170188387650512141, 0.3333333333333333703, 0.3170188387650512141, 0.3333333333333333703, 0.3170188387650512141, 0.3333333333333333703, 0.3170188387650512141, 0.3333333333333333703, 0.3170188387650512141, 0.3333333333333333703, 0.3170188387650512141, 0.3333333333333333703, 0.3170188387650512141, 0.3333333333333333703, 0.3170188387650512141, 0.3333333333333333703, 0.3170188387650512141, 0.3333333333333333703, 0.3170188387650512141, 0.3333333333333333703, 0.3170188387650512141, 0.3333333333333333703, 0.3170188387650512141, 0.3333333333333333703, 0.3170188387650512141, 0.3333333333333333703, 0.3170188387650512141, 0.3333333333333333703, 0.3170188387650512141, 0.3333333333333333703, 0.3170188387650512141, 0.3333333333333333703, 0.3170188387650512141, 0.3333333333333333703, 0.3170188387650512141, 0.3333333333333333703, 0.3170188387650512141, 0.3333333333333333703, 0.3170188387650512141, 0.3333333333333333703, 0.3170188387650512141, 0.3333333333333333703, 0.3170188387650512141, 0.3333333333333333703, 0.3170188387650512141, 0.3333333333333333703, 0.3170188387650512141, 0.3333333333333333703, 0.3170188387650512141, 0.3333333333333333703, 0.3170188387650512141, 0.3333333333333333703, 0.3170188387650512141, 0.3333333333333333703, 0.3170188387650512141, 0.3333333333333333703, 0.3170188387650512141, 0.3333333333333333703, 0.3170188387650512141, 0.3333333333333333703, 0.3170188387650512141, 0.3333333333333333703, 0.3170188387650512141, 0.3333333333333333703, 0.3170188387650512141, 0.3333333333333333703, 0.3170188387650512141, 0.3333333333333333703),
 ( 0.3333333333333333703, 0.3170188387650512141, 0.3333333333333333703, 0.3170188387650512141, 0.3333333333333333703, 0.3170188387650512141, 0.3333333333333333703, 0.3170188387650512141, 0.3333333333333333703, 0.3170188387650512141, 0.3333333333333333703, 0.3170188387650512141, 0.3333333333333333703, 0.3170188387650512141, 0.3333333333333333703, 0.3170188387650512141, 0.3333333333333333703, 0.3170188387650512141, 0.3333333333333333703, 0.3170188387650512141, 0.3333333333333333703, 0.3170188387650512141, 0.3333333333333333703, 0.3170188387650512141, 0.3333333333333333703, 0.3170188387650512141, 0.3333333333333333703, 0.3170188387650512141, 0.3333333333333333703, 0.3170188387650512141, 0.3333333333333333703, 0.3170188387650512141, 0.3333333333333333703, 0.3170188387650512141, 0.3333333333333333703, 0.3170188387650512141, 0.3333333333333333703, 0.3170188387650512141, 0.3333333333333333703, 0.3170188387650512141, 0.3333333333333333703, 0.3170188387650512141, 0.3333333333333333703, 0.3170188387650512141, 0.3333333333333333703, 0.3170188387650512141, 0.3333333333333333703, 0.3170188387650512141, 0.3333333333333333703, 0.3170188387650512141, 0.3333333333333333703, 0.3170188387650512141, 0.3333333333333333703, 0.3170188387650512141, 0.3333333333333333703, 0.3170188387650512141, 0.3333333333333333703, 0.3170188387650512141, 0.3333333333333333703, 0.3170188387650512141, 0.3333333333333333703, 0.3170188387650512141, 0.3333333333333333703, 0.3170188387650512141, 0.3333333333333333703, 0.3170188387650512141, 0.3333333333333333703, 0.3170188387650512141, 0.3333333333333333703, 0.3170188387650512141, 0.3333333333333333703, 0.3170188387650512141, 0.3333333333333333703, 0.3170188387650512141, 0.3333333333333333703, 0.3170188387650512141, 0.3333333333333333703, 0.3170188387650512141, 0.3333333333333333703, 0.3170188387650512141, 0.3333333333333333703, 0.3170188387650512141, 0.3333333333333333703, 0.3170188387650512141, 0.3333333333333333703, 0.3170188387650512141, 0.3333333333333333703, 0.3170188387650512141, 0.3333333333333333703, 0.3170188387650512141, 0.3333333333333333703, 0.3170188387650512141, 0.3333333333333333703, 0.3170188387650512141, 0.3333333333333333703, 0.3170188387650512141, 0.3333333333333333703, 0.3170188387650512141, 0.3333333333333333703, 0.3170188387650512141, 0.3333333333333333703, 0.3170188387650512141, 0.3333333333333333703, 0.3170188387650512141, 0.3333333333333333703, 0.3170188387650512141, 0.3333333333333333703, 0.3170188387650512141, 0.3333333333333333703, 0.3170188387650512141, 0.3333333333333333703, 0.3170188387650512141, 0.3333333333333333703, 0.3170188387650512141, 0.3333333333333333703, 0.3170188387650512141, 0.3333333333333333703, 0.3170188387650512141, 0.3333333333333333703, 0.3170188387650512141, 0.3333333333333333703, 0.3170188387650512141, 0.3333333333333333703, 0.3170188387650512141, 0.3333333333333333703, 0.3170188387650512141, 0.3333333333333333703, 0.3170188387650512141, 0.3333333333333333703, 0.3170188387650512141, 0.3333333333333333703),
 ( 1.000000000000000000, 0.9510565162951535312, 1.000000000000000000, 0.9510565162951535312, 1.000000000000000000, 0.9510565162951535312, 1.000000000000000000, 0.9510565162951535312, 1.000000000000000000, 0.9510565162951535312, 1.000000000000000000, 0.9510565162951535312, 1.000000000000000000, 0.9510565162951535312, 1.000000000000000000, 0.9510565162951535312, 1.000000000000000000, 0.9510565162951535312, 1.000000000000000000, 0.9510565162951535312, 1.000000000000000000, 0.9510565162951535312, 1.000000000000000000, 0.9510565162951535312, 1.000000000000000000, 0.9510565162951535312, 1.000000000000000000, 0.9510565162951535312, 1.000000000000000000, 0.9510565162951535312, 1.000000000000000000, 0.9510565162951535312, 1.000000000000000000, 0.9510565162951535312, 1.000000000000000000, 0.9510565162951535312, 1.000000000000000000, 0.9510565162951535312, 1.000000000000000000, 0.9510565162951535312, 1.000000000000000000, 0.9510565162951535312, 1.000000000000000000, 0.9510565162951535312, 1.000000000000000000, 0.9510565162951535312, 1.000000000000000000, 0.9510565162951535312, 1.000000000000000000, 0.9510565162951535312, 1.000000000000000000, 0.9510565162951535312, 1.000000000000000000, 0.9510565162951535312, 1.000000000000000000, 0.9510565162951535312, 1.000000000000000000, 0.9510565162951535312, 1.000000000000000000, 0.9510565162951535312, 1.000000000000000000, 0.9510565162951535312, 1.000000000000000000, 0.9510565162951535312, 1.000000000000000000, 0.9510565162951535312, 1.000000000000000000, 0.9510565162951535312, 1.000000000000000000, 0.9510565162951535312, 1.000000000000000000, 0.9510565162951535312, 1.000000000000000000, 0.9510565162951535312, 1.000000000000000000, 0.9510565162951535312, 1.000000000000000000, 0.9510565162951535312, 1.000000000000000000, 0.9510565162951535312, 1.000000000000000000, 0.9510565162951535312, 1.000000000000000000, 0.9510565162951535312, 1.000000000000000000, 0.9510565162951535312, 1.000000000000000000, 0.9510565162951535312, 1.000000000000000000, 0.9510565162951535312, 1.000000000000000000, 0.9510565162951535312, 1.000000000000000000, 0.9510565162951535312, 1.000000000000000000, 0.9510565162951535312, 1.000000000000000000, 0.9510565162951535312, 1.000000000000000000, 0.9510565162951535312, 1.000000000000000000, 0.9510565162951535312, 1.000000000000000000, 0.9510565162951535312, 1.000000000000000000, 0.9510565162951535312, 1.000000000000000000, 0.9510565162951535312, 1.000000000000000000, 0.9510565162951535312, 1.000000000000000000, 0.9510565162951535312, 1.000000000000000000, 0.9510565162951535312, 1.000000000000000000, 0.9510565162951535312, 1.000000000000000000, 0.9510565162951535312, 1.000000000000000000, 0.9510565162951535312, 1.000000000000000000, 0.9510565162951535312, 1.000000000000000000, 0.9510565162951535312, 1.000000000000000000, 0.9510565162951535312, 1.000000000000000000, 0.9510565162951535312, 1.000000000000000000, 0.9510565162951535312, 1.000000000000000000) ) ) 
 REPRESENTATION_ITEM ( '' )  SURFACE ( )  );
#5268=CARTESIAN_POINT ( 'NONE',  ( 5.056896391392317724, -9.814260835640970626, 2.648862081921448119 ) ) ;
#5271=CARTESIAN_POINT ( 'NONE',  ( -9.355568503977838901, -4.766900247265280832, 8.399999999999963052 ) ) ;
#5275=CARTESIAN_POINT ( 'NONE',  ( -1.595456901104623348, 10.37818827243067155, -0.6988620819214501623 ) ) ;
#5276=CARTESIAN_POINT ( 'NONE',  ( 7.098671581784200768, 7.027753727702831021, 2.751137918078555789 ) ) ;
#5293=CARTESIAN_POINT ( 'NONE',  ( -9.865911304835474738, -1.562606840307925626, 2.550000000000035350 ) ) ;
#5294=CARTESIAN_POINT ( 'NONE',  ( -7.027753727702738651, -7.098671581784262941, 18.24886208192143044 ) ) ;
#5305=CARTESIAN_POINT ( 'NONE',  ( -5.012215536711506658, 9.837026868206027785, 12.14999999999996305 ) ) ;
#5310=CARTESIAN_POINT ( 'NONE',  ( 10.90442828429183919, 1.727091770866679532, 19.04999999999997939 ) ) ;
#5324=CARTESIAN_POINT ( 'NONE',  ( 8.442910196168311288, 4.355403765523574222, 1.898862081921442790 ) ) ;
#5326=CARTESIAN_POINT ( 'NONE',  ( -7.806708723663830618, -7.806708723663901672, 5.250000000000008882 ) ) ;
#5327=CARTESIAN_POINT ( 'NONE',  ( -7.424621202458789426, 7.424621202458724589, 0.000000000000000000 ) ) ;
#5333=CARTESIAN_POINT ( 'NONE',  ( 9.355568503977840678, 4.766900247265305701, 0.9000000000000119016 ) ) ;
#5337=CARTESIAN_POINT ( 'NONE',  ( 1.612135949262739398, 9.858066664633913234, 11.45113791807854220 ) ) ;
#5338=CARTESIAN_POINT ( 'NONE',  ( -8.486213763410637156, -4.270415729527911708, 1.401137918078568134 ) ) ;
#5351=CARTESIAN_POINT ( 'NONE',  ( -8.900167166472156666, 4.534861676072234893, 11.84999999999997478 ) ) ;
#5352=CARTESIAN_POINT ( 'NONE',  ( -1.533232399700100057, 9.375578539472089190, 13.29886208192143471 ) ) ;
#5353=CARTESIAN_POINT ( 'NONE',  ( -7.071067811865514585, 7.071067811865452413, 0.000000000000000000 ) ) ;
#5359=CARTESIAN_POINT ( 'NONE',  ( -9.355568503977838901, -4.766900247265280832, 14.39999999999996838 ) ) ;
#5362=CARTESIAN_POINT ( 'NONE',  ( 10.89658364409024749, 1.776620879821585897, 11.04886208192144359 ) ) ;
#5367=CARTESIAN_POINT ( 'NONE',  ( 8.464561979789474222, 4.312909747525755400, 9.900000000000019895 ) ) ;
#5373=CARTESIAN_POINT ( 'NONE',  ( 1.513077731352925115, 9.873755945037103743, 10.44886208192141908 ) ) ;
#5375=DIRECTION ( 'NONE',  ( -0.7071067811865510144, 0.7071067811865440200, -6.116266257073745883E-17 ) ) ;
#5376=CARTESIAN_POINT ( 'NONE',  ( -9.814260835641038128, 5.056896391392219137, 10.85113791807856209 ) ) ;
#5381=CARTESIAN_POINT ( 'NONE',  ( 5.012215536711512875, -9.837026868206002916, 4.650000000000027001 ) ) ;
#5383=CARTESIAN_POINT ( 'NONE',  ( -7.098671581784199880, -7.027753727702804376, 16.25113791807856245 ) ) ;
#5384=CARTESIAN_POINT ( 'NONE',  ( 4.490180821391514421, -8.922933199037132113, 0.6511379180785785703 ) ) ;
#5396=CARTESIAN_POINT ( 'NONE',  ( 4.534861676072320158, -8.900167166472096270, 7.649999999999992362 ) ) ;
#5397=CARTESIAN_POINT ( 'NONE',  ( -8.442910196168309511, -4.355403765523546689, 18.39886208192140771 ) ) ;
#5405=CARTESIAN_POINT ( 'NONE',  ( 9.837026868206066865, -5.012215536711395636, 16.35000000000000497 ) ) ;
#5409=CARTESIAN_POINT ( 'NONE',  ( -5.056896391392315948, 9.814260835640997271, 10.14886208192142725 ) ) ;
#5414=CARTESIAN_POINT ( 'NONE',  ( -4.534861676072319270, 8.900167166472122915, 12.14999999999996483 ) ) ;
#5422=CARTESIAN_POINT ( 'NONE',  ( 4.579542530753127672, -8.877401133907065756, 11.64886208192146988 ) ) ;
#5424=CARTESIAN_POINT ( 'NONE',  ( -10.90442828429183919, -1.727091770866654663, 2.550000000000035350 ) ) ;
#5425=CARTESIAN_POINT ( 'NONE',  ( -7.842167650704559456, -7.771249796623176387, 16.25113791807856245 ) ) ;
#5429=CARTESIAN_POINT ( 'NONE',  ( 7.424621202458790314, -7.424621202458697944, 7.500000000000007105 ) ) ;
#5433=CARTESIAN_POINT ( 'NONE',  ( 7.390897758835871301, -7.458344646081617846, 9.501137918078587319 ) ) ;
#5434=CARTESIAN_POINT ( 'NONE',  ( 9.375578539472099848, -1.533232399699987702, 0.2011379180785754783 ) ) ;
#5447=CARTESIAN_POINT ( 'NONE',  ( 8.900167166472154889, -4.534861676072210912, 13.34999999999998188 ) ) ;
#5448=CARTESIAN_POINT ( 'NONE',  ( 9.390499931835536884, -1.439022436064273158, 20.19886208192146526 ) ) ;
#5450=CARTESIAN_POINT ( 'NONE',  ( -9.865911304835474738, -1.562606840307925626, 2.550000000000035794 ) ) ;
#5463=CARTESIAN_POINT ( 'NONE',  ( 9.333916720356675967, 4.809394265263123636, 4.898862081921403266 ) ) ;
#5469=CARTESIAN_POINT ( 'NONE',  ( -6.717514421272238856, 6.717514421272181124, 12.00000000000001066 ) ) ;
#5471=CARTESIAN_POINT ( 'NONE',  ( 9.837026868206066865, -5.012215536711392083, 13.34999999999998188 ) ) ;
#5478=CARTESIAN_POINT ( 'NONE',  ( -1.642561882922479732, 10.37072757624895303, 0.2999999999999669598 ) ) ;
#5479=CARTESIAN_POINT ( 'NONE',  ( -9.355568503977838901, -4.766900247265280832, 2.400000000000013234 ) ) ;
#5487=CARTESIAN_POINT ( 'NONE',  ( -1.642561882922479732, 10.37072757624895303, 0.2999999999999669598 ) ) ;
#5490=CARTESIAN_POINT ( 'NONE',  ( -7.390897758835869524, 7.458344646081644491, 5.001137918078545574 ) ) ;
#5491=CARTESIAN_POINT ( 'NONE',  ( 9.873755945037075321, 1.513077731353044131, 18.05113791807859513 ) ) ;
#5501=CARTESIAN_POINT ( 'NONE',  ( 4.312909747525650594, 8.464561979789532842, 15.60000000000000320 ) ) ;
#5502=CARTESIAN_POINT ( 'NONE',  ( -1.533232399700100057, 9.375578539472098072, 16.29886208192143471 ) ) ;
#5506=CARTESIAN_POINT ( 'NONE',  ( -6.717514421272238856, 6.717514421272176683, 3.000000000000002665 ) ) ;
#5514=CARTESIAN_POINT ( 'NONE',  ( 1.677562661911645714, 10.91227292449346464, 4.448862081921434175 ) ) ;
#5519=CARTESIAN_POINT ( 'NONE',  ( -1.562606840307830591, -9.865911304835481843, 13.95000000000002416 ) ) ;
#5520=CARTESIAN_POINT ( 'NONE',  ( -9.355568503977838901, -4.766900247265280832, 14.39999999999996838 ) ) ;
#5527=CARTESIAN_POINT ( 'NONE',  ( 10.90442828429183919, 1.727091770866679532, 1.049999999999966738 ) ) ;
#5528=CARTESIAN_POINT ( 'NONE',  ( -10.90442828429183919, -1.727091770866655329, 8.549999999999963407 ) ) ;
#5534=CARTESIAN_POINT ( 'NONE',  ( 10.90442828429184274, 1.727091770866679310, 10.05000000000003268 ) ) ;
#5537=CARTESIAN_POINT ( 'NONE',  ( -7.842167650704559456, -7.771249796623180828, 4.251137918078595312 ) ) ;
#5538=CARTESIAN_POINT ( 'NONE',  ( -4.355403765523468529, -8.442910196168352144, 13.10113791807856920 ) ) ;
#5548=CARTESIAN_POINT ( 'NONE',  ( -1.486127417882243895, 9.383039235653816590, 15.29999999999997939 ) ) ;
#5549=CARTESIAN_POINT ( 'NONE',  ( 8.900167166472154889, -4.534861676072210024, 4.350000000000036948 ) ) ;
#5552=CARTESIAN_POINT ( 'NONE',  ( 1.486127417882244783, -9.383039235653791721, 1.800000000000023803 ) ) ;
#5559=CARTESIAN_POINT ( 'NONE',  ( 6.751237864895159646, -6.683790977649239906, 2.498862081921459755 ) ) ;
#5560=CARTESIAN_POINT ( 'NONE',  ( 7.458344646081711105, -7.390897758835778930, 5.498862081921462419 ) ) ;
#5567=CARTESIAN_POINT ( 'NONE',  ( -9.865911304835474738, -1.562606840307925848, 5.549999999999998934 ) ) ;
#5568=CARTESIAN_POINT ( 'NONE',  ( 9.355568503977840678, 4.766900247265305701, 18.90000000000002700 ) ) ;
#5573=CARTESIAN_POINT ( 'NONE',  ( 4.766900247265192903, 9.355568503977902850, 3.599999999999992095 ) ) ;
#5574=CARTESIAN_POINT ( 'NONE',  ( -10.90442828429183919, -1.727091770866654663, 2.550000000000035350 ) ) ;
#5579=CARTESIAN_POINT ( 'NONE',  ( -4.766900247265192014, -9.355568503977876205, 14.10000000000000142 ) ) ;
#5582=CARTESIAN_POINT ( 'NONE',  ( -9.814260835641038128, 5.056896391392219137, 1.851137918078540334 ) ) ;
#5583=CARTESIAN_POINT ( 'NONE',  ( -7.098671581784199880, -7.027753727702804376, 16.25113791807856245 ) ) ;
#5594=CARTESIAN_POINT ( 'NONE',  ( -9.865911304835474738, -1.562606840307925626, 17.55000000000002913 ) ) ;
#5595=CARTESIAN_POINT ( 'NONE',  ( 4.312909747525650594, 8.464561979789541724, 6.599999999999994316 ) ) ;
#5598=CARTESIAN_POINT ( 'NONE',  ( 6.717514421272239744, -6.717514421272154479, 4.500000000000003553 ) ) ;
#5607=CARTESIAN_POINT ( 'NONE',  ( 1.533232399700100945, -9.375578539472067874, 8.798862081921429379 ) ) ;
#5608=CARTESIAN_POINT ( 'NONE',  ( 10.37818827243067510, -1.595456901104499225, 20.19886208192146526 ) ) ;
#5609=CARTESIAN_POINT ( 'NONE',  ( -1.677562661911643938, -10.91227292449344688, 14.94886208192145105 ) ) ;
#5618=CARTESIAN_POINT ( 'NONE',  ( -5.056896391392315948, 9.814260835640997271, 1.148862081921408151 ) ) ;
#5627=CARTESIAN_POINT ( 'NONE',  ( 1.642561882922480621, -10.37072757624891750, 10.80000000000003268 ) ) ;
#5628=CARTESIAN_POINT ( 'NONE',  ( 9.837026868206066865, -5.012215536711391195, 4.350000000000036948 ) ) ;
#5634=CARTESIAN_POINT ( 'NONE',  ( 10.37072757624895836, -1.642561882922356498, 16.19999999999999218 ) ) ;
#5638=CARTESIAN_POINT ( 'NONE',  ( -1.776620879821455556, -10.89658364409025637, 6.951137918078597266 ) ) ;
#5639=CARTESIAN_POINT ( 'NONE',  ( -1.439022436064386845, 9.390499931835526226, 11.30113791807855961 ) ) ;
#5649=CARTESIAN_POINT ( 'NONE',  ( 6.717514421272239744, -6.717514421272154479, 19.50000000000001776 ) ) ;
#5650=CARTESIAN_POINT ( 'NONE',  ( 9.865911304835474738, 1.562606840307949829, 7.050000000000010481 ) ) ;
#5653=CARTESIAN_POINT ( 'NONE',  ( -1.486127417882243895, 9.383039235653816590, 0.2999999999999669598 ) ) ;
#5662=CARTESIAN_POINT ( 'NONE',  ( -8.922933199037192509, 4.490180821391428267, 9.848862081921437195 ) ) ;
#5663=CARTESIAN_POINT ( 'NONE',  ( 1.677562661911645714, 10.91227292449347175, 19.44886208192144039 ) ) ;
#5669=CARTESIAN_POINT ( 'NONE',  ( -1.562606840307830591, -9.865911304835481843, 16.94999999999998863 ) ) ;
#5670=CARTESIAN_POINT ( 'NONE',  ( 10.37818827243067510, -1.595456901104500780, 8.198862081921454603 ) ) ;
#5678=CARTESIAN_POINT ( 'NONE',  ( 9.837026868206066865, -5.012215536711392083, 7.350000000000000533 ) ) ;
#5679=CARTESIAN_POINT ( 'NONE',  ( -9.837026868206066865, 5.012215536711413399, 2.849999999999968114 ) ) ;
#5682=CARTESIAN_POINT ( 'NONE',  ( -9.837026868206070418, 5.012215536711412511, 8.850000000000010303 ) ) ;
#5685=CARTESIAN_POINT ( 'NONE',  ( -10.91227292449344155, -1.677562661911749187, 13.55113791807856316 ) ) ;
#5686=CARTESIAN_POINT ( 'NONE',  ( 8.486213763410640709, 4.270415729527941018, 11.90113791807857702 ) ) ;
#5696=CARTESIAN_POINT ( 'NONE',  ( -4.490180821391513533, 8.922933199037158758, 8.151137918078559252 ) ) ;
#5697=CARTESIAN_POINT ( 'NONE',  ( -7.063212654743466601, -7.063212654743531438, 5.250000000000008882 ) ) ;
#5707=CARTESIAN_POINT ( 'NONE',  ( -7.458344646081709328, 7.390897758835805575, 18.99886208192142334 ) ) ;
#5715=CARTESIAN_POINT ( 'NONE',  ( -10.37818827243067688, 1.595456901104523428, 12.69886208192145816 ) ) ;
#5724=CARTESIAN_POINT ( 'NONE',  ( 4.766900247265192903, 9.355568503977911732, 6.599999999999994316 ) ) ;
#5725=CARTESIAN_POINT ( 'NONE',  ( -1.642561882922479732, 10.37072757624895303, 18.29999999999998295 ) ) ;
#5730=CARTESIAN_POINT ( 'NONE',  ( -1.727091770866549414, -10.90442828429184807, 16.94999999999998863 ) ) ;
#5733=CARTESIAN_POINT ( 'NONE',  ( 1.776620879821457333, 10.89658364409027236, 14.45113791807853509 ) ) ;
#5734=CARTESIAN_POINT ( 'NONE',  ( 4.809394265263009061, 9.333916720356739916, 8.601137918078563871 ) ) ;
#5742=CARTESIAN_POINT ( 'NONE',  ( 8.486213763410640709, 4.270415729527937465, 8.901137918078571687 ) ) ;
#5743=CARTESIAN_POINT ( 'NONE',  ( 8.464561979789474222, 4.312909747525755400, 3.899999999999959055 ) ) ;
#5749=ORIENTED_EDGE ( 'NONE', *, *, #7762, .F. ) ;
#5754=CARTESIAN_POINT ( 'NONE',  ( -9.858066664633883036, -1.612135949262831547, 18.54886208192142405 ) ) ;
#5755=CARTESIAN_POINT ( 'NONE',  ( 4.724406229267374968, 9.377220287599060455, 19.59886208192140700 ) ) ;
#5762=CARTESIAN_POINT ( 'NONE',  ( -4.312909747525649706, -8.464561979789507973, 17.10000000000000497 ) ) ;
#5763=CARTESIAN_POINT ( 'NONE',  ( 1.677562661911645714, 10.91227292449347175, 7.448862081921427070 ) ) ;
#5770=CARTESIAN_POINT ( 'NONE',  ( -1.642561882922479732, 10.37072757624896191, 6.299999999999972289 ) ) ;
#5771=CARTESIAN_POINT ( 'NONE',  ( 10.90442828429183919, 1.727091770866679532, 19.04999999999997939 ) ) ;
#5781=CARTESIAN_POINT ( 'NONE',  ( 10.91227292449344155, 1.677562661911773390, 12.05113791807856671 ) ) ;
#5782=CARTESIAN_POINT ( 'NONE',  ( -1.776620879821455556, -10.89658364409025992, 3.951137918078560851 ) ) ;
#5788=CARTESIAN_POINT ( 'NONE',  ( -7.806708723663830618, -7.806708723663901672, 11.24999999999999467 ) ) ;
#5796=CARTESIAN_POINT ( 'NONE',  ( -4.355403765523468529, -8.442910196168352144, 4.101137918078561206 ) ) ;
#5797=CARTESIAN_POINT ( 'NONE',  ( 1.562606840307832368, 9.865911304835503159, 18.44999999999999218 ) ) ;
#5807=CARTESIAN_POINT ( 'NONE',  ( -4.579542530753125895, 8.877401133907090625, 16.14886208192145389 ) ) ;
#5808=CARTESIAN_POINT ( 'NONE',  ( -6.751237864895158758, 6.683790977649255005, 3.998862081921419342 ) ) ;
#5815=CARTESIAN_POINT ( 'NONE',  ( -10.89658364409024749, -1.776620879821561472, 12.54886208192144004 ) ) ;
#5822=CARTESIAN_POINT ( 'NONE',  ( -9.837026868206066865, 5.012215536711413399, 8.850000000000008527 ) ) ;
#5829=CARTESIAN_POINT ( 'NONE',  ( 4.967534682030706250, -9.859792900771036983, 12.65113791807859123 ) ) ;
#5830=CARTESIAN_POINT ( 'NONE',  ( 10.36326688006723984, -1.689666864740212215, 3.201137918078536426 ) ) ;
#5835=CARTESIAN_POINT ( 'NONE',  ( 4.766900247265192903, 9.355568503977911732, 6.599999999999994316 ) ) ;
#5841=CARTESIAN_POINT ( 'NONE',  ( -7.098671581784199880, -7.027753727702804376, 10.25113791807858021 ) ) ;
#5842=CARTESIAN_POINT ( 'NONE',  ( 4.312909747525650594, 8.464561979789532842, 12.59999999999999964 ) ) ;
#5852=CARTESIAN_POINT ( 'NONE',  ( 9.858066664633883036, 1.612135949262857526, 20.04886208192142050 ) ) ;
#5853=CARTESIAN_POINT ( 'NONE',  ( 1.513077731352925115, 9.873755945037103743, 10.44886208192141908 ) ) ;
#5854=UNCERTAINTY_MEASURE_WITH_UNIT (LENGTH_MEASURE( 1.000000000000000082E-05 ), #5086, 'distance_accuracy_value', 'NONE');
#5861=CARTESIAN_POINT ( 'NONE',  ( -5.056896391392315948, 9.814260835640997271, 10.14886208192142725 ) ) ;
#5867=CARTESIAN_POINT ( 'NONE',  ( 5.056896391392317724, -9.814260835640970626, 2.648862081921448119 ) ) ;
#5876=CARTESIAN_POINT ( 'NONE',  ( 9.333916720356675967, 4.809394265263126300, 16.89886208192141126 ) ) ;
#5878=CARTESIAN_POINT ( 'NONE',  ( -10.91227292449344155, -1.677562661911749187, 10.55113791807857204 ) ) ;
#5879=CARTESIAN_POINT ( 'NONE',  ( 7.842167650704563897, 7.771249796623202144, 2.751137918078555789 ) ) ;
#5883=CARTESIAN_POINT ( 'NONE',  ( 10.90442828429183919, 1.727091770866678422, 4.049999999999988276 ) ) ;
#5889=CARTESIAN_POINT ( 'NONE',  ( 4.490180821391514421, -8.922933199037139218, 3.651137918078570355 ) ) ;
#5890=CARTESIAN_POINT ( 'NONE',  ( 4.312909747525650594, 8.464561979789532842, 15.60000000000000320 ) ) ;
#5904=CARTESIAN_POINT ( 'NONE',  ( 4.579542530753127672, -8.877401133907065756, 17.64886208192141126 ) ) ;
#5905=CARTESIAN_POINT ( 'NONE',  ( -4.270415729527831772, -8.486213763410670907, 9.098862081921437195 ) ) ;
#5919=CARTESIAN_POINT ( 'NONE',  ( 7.771249796623105333, 7.842167650704658932, 1.748862081921432887 ) ) ;
#5928=CARTESIAN_POINT ( 'NONE',  ( 9.390499931835536884, -1.439022436064273158, 2.198862081921450606 ) ) ;
#5930=CARTESIAN_POINT ( 'NONE',  ( 4.766900247265192903, 9.355568503977911732, 6.599999999999994316 ) ) ;
#5931=CARTESIAN_POINT ( 'NONE',  ( -7.842167650704559456, -7.771249796623176387, 7.251137918078588207 ) ) ;
#5935=CARTESIAN_POINT ( 'NONE',  ( -5.012215536711506658, 9.837026868206022456, 6.149999999999980815 ) ) ;
#5943=CARTESIAN_POINT ( 'NONE',  ( 4.490180821391514421, -8.922933199037132113, 12.65113791807859123 ) ) ;
#5944=CARTESIAN_POINT ( 'NONE',  ( -6.683790977649319842, 6.751237864895101026, -0.9988620819214586444 ) ) ;
#5956=CARTESIAN_POINT ( 'NONE',  ( -4.312909747525649706, -8.464561979789507973, 5.099999999999993427 ) ) ;
#5957=CARTESIAN_POINT ( 'NONE',  ( 4.579542530753127672, -8.877401133907065756, 11.64886208192146988 ) ) ;
#5959=CARTESIAN_POINT ( 'NONE',  ( 9.355568503977840678, 4.766900247265305701, 15.90000000000002522 ) ) ;
#5967=ORIENTED_EDGE ( 'NONE', *, *, #8032, .T. ) ;
#5968=CARTESIAN_POINT ( 'NONE',  ( -10.90442828429183919, -1.727091770866654663, 17.55000000000002913 ) ) ;
#5972=CARTESIAN_POINT ( 'NONE',  ( -9.837026868206066865, 5.012215536711413399, 14.84999999999999787 ) ) ;
#5980=CARTESIAN_POINT ( 'NONE',  ( 5.056896391392317724, -9.814260835640970626, 17.64886208192141126 ) ) ;
#5982=CARTESIAN_POINT ( 'NONE',  ( -10.90442828429183919, -1.727091770866655329, 8.549999999999963407 ) ) ;
#5983=CARTESIAN_POINT ( 'NONE',  ( -7.390897758835869524, 7.458344646081637386, 14.00113791807859620 ) ) ;
#5986=CARTESIAN_POINT ( 'NONE',  ( 7.424621202458790314, -7.424621202458697944, 4.500000000000003553 ) ) ;
#5994=CARTESIAN_POINT ( 'NONE',  ( -1.439022436064386845, 9.390499931835535108, 17.30113791807856316 ) ) ;
#5995=CARTESIAN_POINT ( 'NONE',  ( 8.464561979789474222, 4.312909747525755400, 12.90000000000002345 ) ) ;
#6007=CARTESIAN_POINT ( 'NONE',  ( -4.312909747525649706, -8.464561979789499091, 8.099999999999996092 ) ) ;
#6008=CARTESIAN_POINT ( 'NONE',  ( -8.442910196168309511, -4.355403765523546689, 9.398862081921404155 ) ) ;
#6009=CARTESIAN_POINT ( 'NONE',  ( 7.424621202458790314, -7.424621202458697944, 16.50000000000001421 ) ) ;
#6016=CARTESIAN_POINT ( 'NONE',  ( -9.837026868206066865, 5.012215536711416064, 11.84999999999997478 ) ) ;
#6020=CARTESIAN_POINT ( 'NONE',  ( -7.458344646081709328, 7.390897758835804687, 0.9988620819214170110 ) ) ;
#6029=CARTESIAN_POINT ( 'NONE',  ( 1.677562661911645714, 10.91227292449347175, 19.44886208192144039 ) ) ;
#6030=CARTESIAN_POINT ( 'NONE',  ( 4.766900247265192903, 9.355568503977911732, 9.599999999999997868 ) ) ;
#6031=CARTESIAN_POINT ( 'NONE',  ( 4.809394265263009061, 9.333916720356734587, 11.60113791807856742 ) ) ;
#6037=CARTESIAN_POINT ( 'NONE',  ( 7.424621202458790314, -7.424621202458697944, 19.50000000000001776 ) ) ;
#6042=CARTESIAN_POINT ( 'NONE',  ( 8.877401133907127928, -4.579542530753017537, 18.35113791807858519 ) ) ;
#6043=CARTESIAN_POINT ( 'NONE',  ( 4.355403765523470305, 8.442910196168369907, 8.601137918078563871 ) ) ;
#6055=CARTESIAN_POINT ( 'NONE',  ( 1.486127417882244783, -9.383039235653791721, 4.800000000000026468 ) ) ;
#6056=CARTESIAN_POINT ( 'NONE',  ( 4.312909747525650594, 8.464561979789532842, 0.5999999999999894307 ) ) ;
#6057=CARTESIAN_POINT ( 'NONE',  ( -9.837026868206066865, 5.012215536711416064, 11.84999999999997478 ) ) ;
#6067=CARTESIAN_POINT ( 'NONE',  ( 7.806708723663831506, 7.806708723663930982, 12.75000000000000533 ) ) ;
#6071=CARTESIAN_POINT ( 'NONE',  ( 10.89658364409024749, 1.776620879821585897, 2.048862081921423162 ) ) ;
#6082=CARTESIAN_POINT ( 'NONE',  ( 1.689666864740335894, -10.36326688006720786, 17.79886208192143471 ) ) ;
#6084=CARTESIAN_POINT ( 'NONE',  ( -10.90442828429183919, -1.727091770866654663, 2.550000000000035350 ) ) ;
#6085=CARTESIAN_POINT ( 'NONE',  ( 10.36326688006723984, -1.689666864740210883, 18.20113791807854398 ) ) ;
#6092=CARTESIAN_POINT ( 'NONE',  ( 1.642561882922480621, -10.37072757624892638, 1.800000000000023803 ) ) ;
#6095=CARTESIAN_POINT ( 'NONE',  ( 8.486213763410640709, 4.270415729527937465, 17.90113791807857524 ) ) ;
#6096=CARTESIAN_POINT ( 'NONE',  ( 8.486213763410640709, 4.270415729527937465, 8.901137918078571687 ) ) ;
#6112=CARTESIAN_POINT ( 'NONE',  ( -9.865911304835474738, -1.562606840307925626, 11.54999999999998295 ) ) ;
#6113=CARTESIAN_POINT ( 'NONE',  ( 7.027753727702739539, 7.098671581784288698, 16.74886208192143755 ) ) ;
#6128=CARTESIAN_POINT ( 'NONE',  ( 5.056896391392317724, -9.814260835640970626, 11.64886208192146988 ) ) ;
#6132=CARTESIAN_POINT ( 'NONE',  ( -7.063212654743467489, -7.063212654743533214, 5.250000000000008882 ) ) ;
#6138=CARTESIAN_POINT ( 'NONE',  ( -1.513077731352923339, -9.873755945037078874, 5.948862081921430622 ) ) ;
#6141=CARTESIAN_POINT ( 'NONE',  ( 9.377220287599001836, 4.724406229267489543, 17.90113791807857524 ) ) ;
#6146=CARTESIAN_POINT ( 'NONE',  ( -10.90442828429184274, -1.727091770866655773, 5.549999999999998934 ) ) ;
#6151=CARTESIAN_POINT ( 'NONE',  ( -7.098671581784199880, -7.027753727702809705, 13.25113791807857311 ) ) ;
#6152=CARTESIAN_POINT ( 'NONE',  ( -4.490180821391513533, 8.922933199037158758, 8.151137918078559252 ) ) ;
#6163=CARTESIAN_POINT ( 'NONE',  ( 4.766900247265192903, 9.355568503977902850, 0.5999999999999894307 ) ) ;
#6164=CARTESIAN_POINT ( 'NONE',  ( -7.063212654743466601, -7.063212654743531438, 5.250000000000008882 ) ) ;
#6165=CARTESIAN_POINT ( 'NONE',  ( -4.270415729527831772, -8.486213763410670907, 18.09886208192144252 ) ) ;
#6172=CARTESIAN_POINT ( 'NONE',  ( -4.766900247265192014, -9.355568503977876205, 14.10000000000000142 ) ) ;
#6175=CARTESIAN_POINT ( 'NONE',  ( 7.771249796623105333, 7.842167650704653603, 4.748862081921425116 ) ) ;
#6180=CARTESIAN_POINT ( 'NONE',  ( -4.534861676072319270, 8.900167166472117586, 6.149999999999979927 ) ) ;
#6184=PLANE ( 'NONE',  #1277 ) ;
#6187=CARTESIAN_POINT ( 'NONE',  ( 1.533232399700100945, -9.375578539472073203, 11.79886208192143471 ) ) ;
#6190=CARTESIAN_POINT ( 'NONE',  ( 10.37072757624895836, -1.642561882922355831, 1.200000000000034373 ) ) ;
#6191=CARTESIAN_POINT ( 'NONE',  ( 9.377220287599001836, 4.724406229267489543, 14.90113791807857879 ) ) ;
#6197=CARTESIAN_POINT ( 'NONE',  ( 10.37072757624895836, -1.642561882922355609, 7.199999999999984190 ) ) ;
#6201=CARTESIAN_POINT ( 'NONE',  ( 10.36326688006723984, -1.689666864740210883, 9.201137918078538647 ) ) ;
#6202=CARTESIAN_POINT ( 'NONE',  ( -4.490180821391513533, 8.922933199037158758, 5.151137918078567246 ) ) ;
#6213=CARTESIAN_POINT ( 'NONE',  ( 9.865911304835474738, 1.562606840307950051, 13.04999999999999538 ) ) ;
#6214=CARTESIAN_POINT ( 'NONE',  ( 1.562606840307832368, 9.865911304835510265, 0.4499999999999856337 ) ) ;
#6226=CARTESIAN_POINT ( 'NONE',  ( 1.677562661911645714, 10.91227292449346642, 13.44886208192141197 ) ) ;
#6230=CARTESIAN_POINT ( 'NONE',  ( -4.312909747525649706, -8.464561979789499091, 11.09999999999999787 ) ) ;
#6231=CARTESIAN_POINT ( 'NONE',  ( -9.355568503977838901, -4.766900247265279944, 17.39999999999997016 ) ) ;
#6237=CARTESIAN_POINT ( 'NONE',  ( 8.922933199037192509, -4.490180821391404287, 8.348862081921442524 ) ) ;
#6239=CARTESIAN_POINT ( 'NONE',  ( -7.071067811865514585, 7.071067811865452413, 0.000000000000000000 ) ) ;
#6240=CARTESIAN_POINT ( 'NONE',  ( -1.642561882922479732, 10.37072757624896191, 9.299999999999975842 ) ) ;
#6246=CARTESIAN_POINT ( 'NONE',  ( 7.806708723663832394, 7.806708723663930982, 0.7499999999999762412 ) ) ;
#6250=CARTESIAN_POINT ( 'NONE',  ( -7.390897758835869524, 7.458344646081637386, 2.001137918078543354 ) ) ;
#6251=CARTESIAN_POINT ( 'NONE',  ( 4.490180821391514421, -8.922933199037132113, 6.651137918078563693 ) ) ;
#6260=CARTESIAN_POINT ( 'NONE',  ( -6.717514421272238856, 6.717514421272180236, 15.00000000000001421 ) ) ;
#6261=CARTESIAN_POINT ( 'NONE',  ( 8.900167166472154889, -4.534861676072210912, 1.350000000000015188 ) ) ;
#6274=STYLED_ITEM ( 'NONE', ( #3490 ), #206 ) ;
#6276=CARTESIAN_POINT ( 'NONE',  ( 10.89658364409024749, 1.776620879821585897, 8.048862081921450695 ) ) ;
#6280=CARTESIAN_POINT ( 'NONE',  ( -4.312909747525649706, -8.464561979789507973, 5.099999999999993427 ) ) ;
#6281=CARTESIAN_POINT ( 'NONE',  ( -7.458344646081709328, 7.390897758835804687, 0.9988620819214170110 ) ) ;
#6290=CARTESIAN_POINT ( 'NONE',  ( -1.727091770866549414, -10.90442828429184274, 7.950000000000040146 ) ) ;
#6293=AXIS2_PLACEMENT_3D ( 'NONE', #3144, #9469, #6337 ) ;
#6294=SURFACE_STYLE_FILL_AREA ( #3308 ) ;
#6297=CARTESIAN_POINT ( 'NONE',  ( 10.37072757624895836, -1.642561882922355609, 10.19999999999998685 ) ) ;
#6301=CARTESIAN_POINT ( 'NONE',  ( -1.595456901104623348, 10.37818827243067155, 5.301137918078554279 ) ) ;
#6302=CARTESIAN_POINT ( 'NONE',  ( -4.967534682030703586, 9.859792900771061852, -0.8488620819214613977 ) ) ;
#6313=CARTESIAN_POINT ( 'NONE',  ( 8.464561979789474222, 4.312909747525755400, 15.90000000000002522 ) ) ;
#6314=CARTESIAN_POINT ( 'NONE',  ( -9.383039235653820143, 1.486127417882155521, 8.700000000000041922 ) ) ;
#6316=CARTESIAN_POINT ( 'NONE',  ( 1.562606840307832146, 9.865911304835508489, 0.4499999999999857447 ) ) ;
#6320=( BOUNDED_CURVE ( )  B_SPLINE_CURVE ( 2, ( #3335, #8030, #5653, #6316, #6367, #125, #4885, #960, #1537, #7880, #9545, #859, #5552, #7255, #177, #4733, #1633, #5450, #9392, #4683, #5506, #9449, #7984, #806, #911, #8761, #4779, #3955, #7930, #2452, #5598, #1689, #4831, #3198, #6280, #6132, #4649, #5567, #3088, #1448, #2317, #6180, #9308, #2419, #7803, #4029, #2987, #6333, #725, #4698, #7751, #2221, #771, #10123, #10071, #3918, #7124, #40, #7016, #3973, #9513, #10173, #8728, #1649, #7894, #877, #5367, #4796, #3873, #8523, #3824, #9357, #7949, #4597, #6230, #2267, #9407, #672, #6961, #3040, #5469, #5414, #8572, #8629, #819, #7845, #1496, #1551, #7063, #10226, #3136, #9465, #2367, #5519, #8678, #1600, #4749, #1703, #976, #2572, #7223, #5001, #90, #141, #300, #8147, #8883, #4124, #6435, #1851, #1127, #7273, #8990, #5669, #5762, #8101, #7325, #6383, #7173, #8934, #8785, #199, #4848, #9664, #6581, #9618, #1030, #7373, #4176, #3351, #3442 ),
 .UNSPECIFIED., .F., .T. ) 
 B_SPLINE_CURVE_WITH_KNOTS ( ( 3, 2, 2, 2, 2, 2, 2, 2, 2, 2, 2, 2, 2, 2, 2, 2, 2, 2, 2, 2, 2, 2, 2, 2, 2, 2, 2, 2, 2, 2, 2, 2, 2, 2, 2, 2, 2, 2, 2, 2, 2, 2, 2, 2, 2, 2, 2, 2, 2, 2, 2, 2, 2, 2, 2, 2, 2, 2, 2, 2, 2, 2, 2, 2, 2, 3 ),
 ( 0.000000000000000000, 0.01428571428571428527, 0.02857142857142857054, 0.04285714285714285060, 0.05714285714285714107, 0.07142857142857142461, 0.08571428571428570120, 0.1000000000000000056, 0.1142857142857142821, 0.1285714285714285587, 0.1428571428571428492, 0.1571428571428571397, 0.1714285714285714024, 0.1857142857142857206, 0.2000000000000000111, 0.2142857142857142738, 0.2285714285714285643, 0.2428571428571428548, 0.2571428571428571175, 0.2714285714285714080, 0.2857142857142856984, 0.2999999999999999889, 0.3142857142857142794, 0.3285714285714285698, 0.3428571428571428048, 0.3571428571428571508, 0.3714285714285714413, 0.3857142857142857317, 0.4000000000000000222, 0.4142857142857143127, 0.4285714285714285476, 0.4428571428571428381, 0.4571428571428571286, 0.4714285714285714191, 0.4857142857142857095, 0.5000000000000000000, 0.5142857142857142350, 0.5285714285714285809, 0.5428571428571428159, 0.5571428571428571619, 0.5714285714285713969, 0.5857142857142857428, 0.5999999999999999778, 0.6142857142857143238, 0.6285714285714285587, 0.6428571428571429047, 0.6571428571428571397, 0.6714285714285713746, 0.6857142857142856096, 0.6999999999999999556, 0.7142857142857143016, 0.7285714285714285365, 0.7428571428571428825, 0.7571428571428571175, 0.7714285714285714635, 0.7857142857142856984, 0.8000000000000000444, 0.8142857142857143904, 0.8285714285714286254, 0.8428571428571428603, 0.8571428571428570953, 0.8714285714285714413, 0.8857142857142856762, 0.9000000000000000222, 0.9142857142857142572, 0.9285714285714286031 ),
 .UNSPECIFIED. ) 
 CURVE ( )  GEOMETRIC_REPRESENTATION_ITEM ( )  RATIONAL_B_SPLINE_CURVE ( ( 1.000000000000000000, 0.9510565162951535312, 1.000000000000000000, 0.9510565162951535312, 1.000000000000000000, 0.9510565162951535312, 1.000000000000000000, 0.9510565162951535312, 1.000000000000000000, 0.9510565162951535312, 1.000000000000000000, 0.9510565162951535312, 1.000000000000000000, 0.9510565162951535312, 1.000000000000000000, 0.9510565162951535312, 1.000000000000000000, 0.9510565162951535312, 1.000000000000000000, 0.9510565162951535312, 1.000000000000000000, 0.9510565162951535312, 1.000000000000000000, 0.9510565162951535312, 1.000000000000000000, 0.9510565162951535312, 1.000000000000000000, 0.9510565162951535312, 1.000000000000000000, 0.9510565162951535312, 1.000000000000000000, 0.9510565162951535312, 1.000000000000000000, 0.9510565162951535312, 1.000000000000000000, 0.9510565162951535312, 1.000000000000000000, 0.9510565162951535312, 1.000000000000000000, 0.9510565162951535312, 1.000000000000000000, 0.9510565162951535312, 1.000000000000000000, 0.9510565162951535312, 1.000000000000000000, 0.9510565162951535312, 1.000000000000000000, 0.9510565162951535312, 1.000000000000000000, 0.9510565162951535312, 1.000000000000000000, 0.9510565162951535312, 1.000000000000000000, 0.9510565162951535312, 1.000000000000000000, 0.9510565162951535312, 1.000000000000000000, 0.9510565162951535312, 1.000000000000000000, 0.9510565162951535312, 1.000000000000000000, 0.9510565162951535312, 1.000000000000000000, 0.9510565162951535312, 1.000000000000000000, 0.9510565162951535312, 1.000000000000000000, 0.9510565162951535312, 1.000000000000000000, 0.9510565162951535312, 1.000000000000000000, 0.9510565162951535312, 1.000000000000000000, 0.9510565162951535312, 1.000000000000000000, 0.9510565162951535312, 1.000000000000000000, 0.9510565162951535312, 1.000000000000000000, 0.9510565162951535312, 1.000000000000000000, 0.9510565162951535312, 1.000000000000000000, 0.9510565162951535312, 1.000000000000000000, 0.9510565162951535312, 1.000000000000000000, 0.9510565162951535312, 1.000000000000000000, 0.9510565162951535312, 1.000000000000000000, 0.9510565162951535312, 1.000000000000000000, 0.9510565162951535312, 1.000000000000000000, 0.9510565162951535312, 1.000000000000000000, 0.9510565162951535312, 1.000000000000000000, 0.9510565162951535312, 1.000000000000000000, 0.9510565162951535312, 1.000000000000000000, 0.9510565162951535312, 1.000000000000000000, 0.9510565162951535312, 1.000000000000000000, 0.9510565162951535312, 1.000000000000000000, 0.9510565162951535312, 1.000000000000000000, 0.9510565162951535312, 1.000000000000000000, 0.9510565162951535312, 1.000000000000000000, 0.9510565162951535312, 1.000000000000000000, 0.9510565162951535312, 1.000000000000000000, 0.9510565162951535312, 1.000000000000000000, 0.9510565162951535312, 1.000000000000000000, 0.9510565162951535312, 1.000000000000000000, 0.9510565162951535312, 1.000000000000000000, 0.9510565162951535312, 1.000000000000000000, 0.9510565162951535312, 1.000000000000000000 ) ) 
 REPRESENTATION_ITEM ( '' )  );
#6322=EDGE_LOOP ( 'NONE', ( #1772, #5749 ) ) ;
#6325=CARTESIAN_POINT ( 'NONE',  ( 9.859792900771104485, -4.967534682030585458, 20.34886208192140700 ) ) ;
#6327=CARTESIAN_POINT ( 'NONE',  ( -7.771249796623103556, -7.842167650704634063, 9.248862081921457090 ) ) ;
#6333=CARTESIAN_POINT ( 'NONE',  ( 9.865911304835478290, 1.562606840307950051, 7.050000000000010481 ) ) ;
#6334=CARTESIAN_POINT ( 'NONE',  ( 9.355568503977840678, 4.766900247265305701, 15.90000000000002522 ) ) ;
#6337=DIRECTION ( 'NONE',  ( 0.7071067811865505703, -0.7071067811865444641, 0.000000000000000000 ) ) ;
#6341=CARTESIAN_POINT ( 'NONE',  ( -7.806708723663830618, -7.806708723663906113, 2.249999999999986233 ) ) ;
#6342=CARTESIAN_POINT ( 'NONE',  ( 4.766900247265192903, 9.355568503977902850, 0.5999999999999894307 ) ) ;
#6345=( NAMED_UNIT ( * ) PLANE_ANGLE_UNIT ( ) SI_UNIT ( $, .RADIAN. ) );
#6349=CARTESIAN_POINT ( 'NONE',  ( -9.355568503977838901, -4.766900247265279944, 17.39999999999997016 ) ) ;
#6352=CARTESIAN_POINT ( 'NONE',  ( 7.390897758835871301, -7.458344646081618734, 0.5011379180785839882 ) ) ;
#6353=CARTESIAN_POINT ( 'NONE',  ( -9.873755945037078874, -1.513077731353019706, 13.55113791807856316 ) ) ;
#6363=CARTESIAN_POINT ( 'NONE',  ( 8.900167166472154889, -4.534861676072210912, 19.34999999999996945 ) ) ;
#6364=CARTESIAN_POINT ( 'NONE',  ( -6.717514421272238856, 6.717514421272181124, 6.000000000000005329 ) ) ;
#6367=CARTESIAN_POINT ( 'NONE',  ( 4.312909747525650594, 8.464561979789532842, 0.5999999999999894307 ) ) ;
#6376=CARTESIAN_POINT ( 'NONE',  ( 4.270415729527831772, 8.486213763410688671, 1.598862081921434308 ) ) ;
#6377=CARTESIAN_POINT ( 'NONE',  ( 9.333916720356675967, 4.809394265263123636, 13.89886208192141126 ) ) ;
#6383=CARTESIAN_POINT ( 'NONE',  ( -9.865911304835474738, -1.562606840307925626, 17.55000000000002913 ) ) ;
#6384=CARTESIAN_POINT ( 'NONE',  ( 10.37072757624895836, -1.642561882922355831, 19.19999999999999574 ) ) ;
#6392=CARTESIAN_POINT ( 'NONE',  ( -10.90442828429183919, -1.727091770866654663, 11.54999999999998295 ) ) ;
#6393=CARTESIAN_POINT ( 'NONE',  ( -9.837026868206066865, 5.012215536711413399, 8.850000000000008527 ) ) ;
#6399=CARTESIAN_POINT ( 'NONE',  ( 7.806708723663832394, 7.806708723663930982, 12.75000000000000355 ) ) ;
#6403=CARTESIAN_POINT ( 'NONE',  ( 1.595456901104624459, -10.37818827243064490, 6.801137918078597799 ) ) ;
#6404=CARTESIAN_POINT ( 'NONE',  ( 9.873755945037075321, 1.513077731353044131, 12.05113791807856671 ) ) ;
#6414=CARTESIAN_POINT ( 'NONE',  ( -7.063212654743466601, -7.063212654743531438, 17.25000000000003553 ) ) ;
#6415=CARTESIAN_POINT ( 'NONE',  ( -9.865911304835474738, -1.562606840307925626, 5.549999999999999822 ) ) ;
#6427=CARTESIAN_POINT ( 'NONE',  ( -8.922933199037192509, 4.490180821391424715, 6.848862081921446077 ) ) ;
#6428=CARTESIAN_POINT ( 'NONE',  ( -1.689666864740335228, 10.36326688006723273, 19.29886208192143471 ) ) ;
#6435=CARTESIAN_POINT ( 'NONE',  ( 9.383039235653818366, -1.486127417882131097, 16.19999999999999218 ) ) ;
#6436=CARTESIAN_POINT ( 'NONE',  ( -1.677562661911643938, -10.91227292449344688, 11.94886208192145993 ) ) ;
#6441=AXIS2_PLACEMENT_3D ( 'NONE', #5353, #2304, #8556 ) ;
#6446=CARTESIAN_POINT ( 'NONE',  ( 4.766900247265192903, 9.355568503977902850, 12.59999999999999964 ) ) ;
#6447=CARTESIAN_POINT ( 'NONE',  ( -10.37072757624895836, 1.642561882922381145, 8.700000000000041922 ) ) ;
#6452=CARTESIAN_POINT ( 'NONE',  ( 9.355568503977840678, 4.766900247265305701, 9.900000000000019895 ) ) ;
#6456=CARTESIAN_POINT ( 'NONE',  ( -7.842167650704559456, -7.771249796623180828, 13.25113791807857311 ) ) ;
#6457=CARTESIAN_POINT ( 'NONE',  ( 8.486213763410640709, 4.270415729527937465, 14.90113791807857879 ) ) ;
#6468=CARTESIAN_POINT ( 'NONE',  ( -8.486213763410637156, -4.270415729527911708, 10.40113791807857524 ) ) ;
#6469=CARTESIAN_POINT ( 'NONE',  ( -1.562606840307830591, -9.865911304835478290, 10.95000000000000462 ) ) ;
#6475=DIRECTION ( 'NONE',  ( 0.7071067811865510144, -0.7071067811865440200, 0.000000000000000000 ) ) ;
#6477=CARTESIAN_POINT ( 'NONE',  ( -1.533232399700100057, 9.375578539472094519, 10.29886208192143293 ) ) ;
#6478=CARTESIAN_POINT ( 'NONE',  ( -4.724406229267374968, -9.377220287599040915, 15.09886208192144430 ) ) ;
#6487=CARTESIAN_POINT ( 'NONE',  ( -7.458344646081709328, 7.390897758835804687, 9.998862081921425116 ) ) ;
#6488=ORIENTED_EDGE ( 'NONE', *, *, #1414, .T. ) ;
#6494=CARTESIAN_POINT ( 'NONE',  ( -5.012215536711506658, 9.837026868206027785, 9.150000000000003908 ) ) ;
#6495=CARTESIAN_POINT ( 'NONE',  ( 10.90442828429183919, 1.727091770866679532, 13.04999999999999538 ) ) ;
#6498=CARTESIAN_POINT ( 'NONE',  ( -9.355568503977838901, -4.766900247265280832, 14.39999999999996838 ) ) ;
#6501=CARTESIAN_POINT ( 'NONE',  ( 4.809394265263009061, 9.333916720356739916, 14.60113791807856920 ) ) ;
#6502=CARTESIAN_POINT ( 'NONE',  ( -7.390897758835869524, 7.458344646081644491, 8.001137918078546463 ) ) ;
#6512=CARTESIAN_POINT ( 'NONE',  ( -7.098671581784199880, -7.027753727702804376, 7.251137918078588207 ) ) ;
#6513=CARTESIAN_POINT ( 'NONE',  ( -7.063212654743466601, -7.063212654743534991, 2.249999999999986233 ) ) ;
#6524=CARTESIAN_POINT ( 'NONE',  ( -4.312909747525649706, -8.464561979789507973, 2.099999999999990763 ) ) ;
#6525=CARTESIAN_POINT ( 'NONE',  ( -4.724406229267374968, -9.377220287599040915, 18.09886208192144252 ) ) ;
#6533=CARTESIAN_POINT ( 'NONE',  ( -4.724406229267374968, -9.377220287599040915, 6.098862081921437195 ) ) ;
#6541=CARTESIAN_POINT ( 'NONE',  ( -10.37072757624895836, 1.642561882922381145, 8.700000000000041922 ) ) ;
#6542=CARTESIAN_POINT ( 'NONE',  ( 7.806708723663831506, 7.806708723663931870, 18.74999999999998934 ) ) ;
#6549=CARTESIAN_POINT ( 'NONE',  ( -4.967534682030703586, 9.859792900771061852, 11.15113791807855215 ) ) ;
#6550=CARTESIAN_POINT ( 'NONE',  ( 10.91227292449344155, 1.677562661911773390, 0.05113791807855379290 ) ) ;
#6554=CARTESIAN_POINT ( 'NONE',  ( 9.837026868206066865, -5.012215536711391195, 10.35000000000002274 ) ) ;
#6561=CARTESIAN_POINT ( 'NONE',  ( -6.683790977649319842, 6.751237864895101026, 5.001137918078545574 ) ) ;
#6562=CARTESIAN_POINT ( 'NONE',  ( -8.464561979789474222, -4.312909747525728754, 11.39999999999996660 ) ) ;
#6572=CARTESIAN_POINT ( 'NONE',  ( -8.922933199037192509, 4.490180821391428267, 18.84886208192146029 ) ) ;
#6573=CARTESIAN_POINT ( 'NONE',  ( -9.858066664633883036, -1.612135949262833323, 3.548862081921419609 ) ) ;
#6581=CARTESIAN_POINT ( 'NONE',  ( 4.312909747525650594, 8.464561979789532842, 18.60000000000000497 ) ) ;
#6582=CARTESIAN_POINT ( 'NONE',  ( -10.89658364409024749, -1.776620879821559917, 6.548862081921412504 ) ) ;
#6590=CARTESIAN_POINT ( 'NONE',  ( -7.806708723663830618, -7.806708723663906113, 8.250000000000028422 ) ) ;
#6599=CARTESIAN_POINT ( 'NONE',  ( 9.355568503977840678, 4.766900247265305701, 0.9000000000000119016 ) ) ;
#6600=CARTESIAN_POINT ( 'NONE',  ( 10.91227292449344155, 1.677562661911774944, 9.051137918078573819 ) ) ;
#6603=CARTESIAN_POINT ( 'NONE',  ( -9.837026868206066865, 5.012215536711416064, 5.849999999999989875 ) ) ;
#6609=CARTESIAN_POINT ( 'NONE',  ( -4.355403765523468529, -8.442910196168346815, 7.101137918078564759 ) ) ;
#6610=CARTESIAN_POINT ( 'NONE',  ( 4.355403765523470305, 8.442910196168369907, -0.3988620819214416247 ) ) ;
#6622=CARTESIAN_POINT ( 'NONE',  ( 1.513077731352925115, 9.873755945037103743, 19.44886208192144039 ) ) ;
#6623=CARTESIAN_POINT ( 'NONE',  ( 1.513077731352925115, 9.873755945037098414, 4.448862081921434175 ) ) ;
#6632=CARTESIAN_POINT ( 'NONE',  ( -7.771249796623103556, -7.842167650704634063, 9.248862081921457090 ) ) ;
#6638=CARTESIAN_POINT ( 'NONE',  ( -9.355568503977838901, -4.766900247265279944, 17.39999999999997016 ) ) ;
#6645=CARTESIAN_POINT ( 'NONE',  ( 9.858066664633883036, 1.612135949262857526, 2.048862081921423162 ) ) ;
#6647=CARTESIAN_POINT ( 'NONE',  ( -4.809394265263009061, -9.333916720356723928, 13.10113791807856920 ) ) ;
#6648=CARTESIAN_POINT ( 'NONE',  ( 4.967534682030706250, -9.859792900771042312, 3.651137918078570355 ) ) ;
#6652=CARTESIAN_POINT ( 'NONE',  ( -4.766900247265192014, -9.355568503977876205, 5.099999999999993427 ) ) ;
#6658=CARTESIAN_POINT ( 'NONE',  ( 1.612135949262739398, 9.858066664633913234, 2.451137918078564848 ) ) ;
#6659=CARTESIAN_POINT ( 'NONE',  ( 1.486127417882244783, -9.383039235653791721, 16.80000000000003624 ) ) ;
#6668=CARTESIAN_POINT ( 'NONE',  ( 6.751237864895159646, -6.683790977649233689, 17.49886208192142689 ) ) ;
#6669=CARTESIAN_POINT ( 'NONE',  ( 9.390499931835536884, -1.439022436064273158, 5.198862081921453715 ) ) ;
#6683=CARTESIAN_POINT ( 'NONE',  ( 9.355568503977840678, 4.766900247265305701, 15.90000000000002522 ) ) ;
#6692=CARTESIAN_POINT ( 'NONE',  ( 9.859792900771104485, -4.967534682030585458, 20.34886208192140700 ) ) ;
#6693=CARTESIAN_POINT ( 'NONE',  ( 5.012215536711511987, -9.837026868205999364, 4.650000000000026112 ) ) ;
#6694=CARTESIAN_POINT ( 'NONE',  ( -9.814260835641038128, 5.056896391392219137, 1.851137918078540334 ) ) ;
#6698=CARTESIAN_POINT ( 'NONE',  ( 5.012215536711511987, -9.837026868205999364, 4.650000000000026112 ) ) ;
#6704=( GEOMETRIC_REPRESENTATION_CONTEXT ( 3 ) GLOBAL_UNCERTAINTY_ASSIGNED_CONTEXT ( ( #4943 ) ) GLOBAL_UNIT_ASSIGNED_CONTEXT ( ( #9420, #10136, #8428 ) ) REPRESENTATION_CONTEXT ( 'NONE', 'WORKASPACE' ) );
#6706=CARTESIAN_POINT ( 'NONE',  ( -8.486213763410637156, -4.270415729527911708, 13.40113791807857702 ) ) ;
#6707=CARTESIAN_POINT ( 'NONE',  ( -4.534861676072319270, 8.900167166472121139, 12.14999999999996305 ) ) ;
#6719=CARTESIAN_POINT ( 'NONE',  ( -1.513077731352923339, -9.873755945037078874, 14.94886208192145105 ) ) ;
#6720=CARTESIAN_POINT ( 'NONE',  ( 1.533232399700100945, -9.375578539472067874, 5.798862081921429379 ) ) ;
#6721=CARTESIAN_POINT ( 'NONE',  ( -1.642561882922479732, 10.37072757624895303, 15.29999999999997939 ) ) ;
#6733=CARTESIAN_POINT ( 'NONE',  ( -4.724406229267374968, -9.377220287599046245, 3.098862081921434974 ) ) ;
#6740=CARTESIAN_POINT ( 'NONE',  ( -5.056896391392315948, 9.814260835640997271, 16.14886208192145389 ) ) ;
#6742=CARTESIAN_POINT ( 'NONE',  ( 10.90442828429183919, 1.727091770866679310, 7.050000000000010481 ) ) ;
#6743=CARTESIAN_POINT ( 'NONE',  ( -1.776620879821455556, -10.89658364409025637, 9.951137918078590161 ) ) ;
#6750=CARTESIAN_POINT ( 'NONE',  ( -10.37072757624895836, 1.642561882922381145, 8.700000000000041922 ) ) ;
#6758=CARTESIAN_POINT ( 'NONE',  ( -4.490180821391513533, 8.922933199037158758, 17.15113791807853616 ) ) ;
#6759=CARTESIAN_POINT ( 'NONE',  ( 9.383039235653818366, -1.486127417882130208, 19.19999999999999574 ) ) ;
#6771=CARTESIAN_POINT ( 'NONE',  ( -10.90442828429183919, -1.727091770866654663, 2.550000000000035350 ) ) ;
#6773=CARTESIAN_POINT ( 'NONE',  ( -9.383039235653820143, 1.486127417882155299, 2.700000000000035705 ) ) ;
#6774=CARTESIAN_POINT ( 'NONE',  ( -7.027753727702738651, -7.098671581784262941, 9.248862081921457090 ) ) ;
#6777=CARTESIAN_POINT ( 'NONE',  ( 5.012215536711511987, -9.837026868205999364, 10.65000000000000924 ) ) ;
#6788=CARTESIAN_POINT ( 'NONE',  ( -10.37072757624895836, 1.642561882922380034, 14.69999999999999041 ) ) ;
#6793=CARTESIAN_POINT ( 'NONE',  ( -7.424621202458789426, 7.424621202458724589, 18.00000000000001421 ) ) ;
#6800=DIRECTION ( 'NONE',  ( -0.7071067811865501263, 0.7071067811865450192, 0.000000000000000000 ) ) ;
#6803=CARTESIAN_POINT ( 'NONE',  ( -1.689666864740335228, 10.36326688006723273, 19.29886208192143471 ) ) ;
#6805=CARTESIAN_POINT ( 'NONE',  ( -5.012215536711506658, 9.837026868206027785, 9.150000000000003908 ) ) ;
#6806=CARTESIAN_POINT ( 'NONE',  ( -9.377220287598998283, -4.724406229267462898, 10.40113791807857524 ) ) ;
#6810=CARTESIAN_POINT ( 'NONE',  ( 9.333916720356675967, 4.809394265263123636, 1.898862081921442790 ) ) ;
#6818=CARTESIAN_POINT ( 'NONE',  ( -8.486213763410637156, -4.270415729527911708, 16.40113791807857524 ) ) ;
#6819=CARTESIAN_POINT ( 'NONE',  ( -1.439022436064386845, 9.390499931835535108, 5.301137918078554279 ) ) ;
#6828=CARTESIAN_POINT ( 'NONE',  ( 10.90442828429183919, 1.727091770866679532, 1.049999999999966738 ) ) ;
#6829=CARTESIAN_POINT ( 'NONE',  ( 6.717514421272239744, -6.717514421272154479, 10.50000000000000888 ) ) ;
#6830=CARTESIAN_POINT ( 'NONE',  ( 8.442910196168311288, 4.355403765523574222, 19.89886208192141481 ) ) ;
#6831=CARTESIAN_POINT ( 'NONE',  ( 9.355568503977840678, 4.766900247265305701, 12.90000000000002345 ) ) ;
#6840=CARTESIAN_POINT ( 'NONE',  ( 9.837026868206066865, -5.012215536711392083, 19.34999999999996945 ) ) ;
#6845=CARTESIAN_POINT ( 'NONE',  ( 1.642561882922480621, -10.37072757624892638, 16.80000000000003624 ) ) ;
#6857=CARTESIAN_POINT ( 'NONE',  ( -9.859792900771106261, 4.967534682030607662, 15.84886208192146739 ) ) ;
#6858=CARTESIAN_POINT ( 'NONE',  ( 10.37072757624895836, -1.642561882922355831, 1.200000000000034373 ) ) ;
#6859=CARTESIAN_POINT ( 'NONE',  ( 7.842167650704563897, 7.771249796623202144, 17.75113791807856245 ) ) ;
#6862=CARTESIAN_POINT ( 'NONE',  ( 10.90442828429183919, 1.727091770866679532, 16.04999999999995808 ) ) ;
#6864=CARTESIAN_POINT ( 'NONE',  ( -9.837026868206070418, 5.012215536711412511, 2.849999999999968114 ) ) ;
#6869=CARTESIAN_POINT ( 'NONE',  ( -7.390897758835869524, 7.458344646081644491, -0.9988620819214586444 ) ) ;
#6870=CARTESIAN_POINT ( 'NONE',  ( 7.098671581784200768, 7.027753727702831021, 8.751137918078539357 ) ) ;
#6882=CARTESIAN_POINT ( 'NONE',  ( 1.642561882922480621, -10.37072757624892638, 1.800000000000023803 ) ) ;
#6883=CARTESIAN_POINT ( 'NONE',  ( -4.312909747525649706, -8.464561979789499091, 11.09999999999999787 ) ) ;
#6884=CARTESIAN_POINT ( 'NONE',  ( 4.579542530753127672, -8.877401133907071085, 14.64886208192141659 ) ) ;
#6894=CARTESIAN_POINT ( 'NONE',  ( 1.642561882922480621, -10.37072757624892638, 13.80000000000003446 ) ) ;
#6898=CARTESIAN_POINT ( 'NONE',  ( -9.859792900771106261, 4.967534682030611215, 9.848862081921437195 ) ) ;
#6909=CARTESIAN_POINT ( 'NONE',  ( -8.442910196168309511, -4.355403765523544024, 12.39886208192140948 ) ) ;
#6911=CARTESIAN_POINT ( 'NONE',  ( -7.424621202458789426, 7.424621202458724589, 6.000000000000005329 ) ) ;
#6912=CARTESIAN_POINT ( 'NONE',  ( -4.809394265263009061, -9.333916720356723928, 13.10113791807856920 ) ) ;
#6917=CARTESIAN_POINT ( 'NONE',  ( -7.806708723663831506, -7.806708723663907001, 2.249999999999986677 ) ) ;
#6921=CARTESIAN_POINT ( 'NONE',  ( 7.098671581784200768, 7.027753727702823916, 14.75113791807856956 ) ) ;
#6922=CARTESIAN_POINT ( 'NONE',  ( -6.683790977649319842, 6.751237864895094809, 2.001137918078543354 ) ) ;
#6939=CARTESIAN_POINT ( 'NONE',  ( -8.464561979789474222, -4.312909747525729642, 8.399999999999963052 ) ) ;
#6940=CARTESIAN_POINT ( 'NONE',  ( -9.390499931835536884, 1.439022436064298249, 12.69886208192145816 ) ) ;
#6951=CARTESIAN_POINT ( 'NONE',  ( -10.90442828429183919, -1.727091770866654663, 14.55000000000000249 ) ) ;
#6955=CARTESIAN_POINT ( 'NONE',  ( -5.056896391392315948, 9.814260835640997271, 7.148862081921437017 ) ) ;
#6961=CARTESIAN_POINT ( 'NONE',  ( -9.383039235653820143, 1.486127417882154411, 11.69999999999998863 ) ) ;
#6968=CARTESIAN_POINT ( 'NONE',  ( -7.027753727702738651, -7.098671581784262941, 12.24886208192144998 ) ) ;
#6971=CARTESIAN_POINT ( 'NONE',  ( -10.91227292449344155, -1.677562661911749187, 10.55113791807857204 ) ) ;
#6978=CARTESIAN_POINT ( 'NONE',  ( 7.424621202458790314, -7.424621202458697944, 4.500000000000003553 ) ) ;
#6981=CARTESIAN_POINT ( 'NONE',  ( -9.814260835641038128, 5.056896391392221801, 4.851137918078532785 ) ) ;
#6982=CARTESIAN_POINT ( 'NONE',  ( 1.612135949262739398, 9.858066664633913234, 2.451137918078564848 ) ) ;
#6996=CARTESIAN_POINT ( 'NONE',  ( 7.063212654743467489, 7.063212654743559860, 3.749999999999997335 ) ) ;
#6997=CARTESIAN_POINT ( 'NONE',  ( -8.922933199037192509, 4.490180821391428267, 18.84886208192146029 ) ) ;
#7004=CARTESIAN_POINT ( 'NONE',  ( -4.766900247265192014, -9.355568503977876205, 17.10000000000000497 ) ) ;
#7009=CARTESIAN_POINT ( 'NONE',  ( -7.771249796623103556, -7.842167650704634063, 12.24886208192144998 ) ) ;
#7016=CARTESIAN_POINT ( 'NONE',  ( -9.383039235653820143, 1.486127417882155521, 8.700000000000041922 ) ) ;
#7023=CARTESIAN_POINT ( 'NONE',  ( -4.270415729527831772, -8.486213763410670907, 6.098862081921437195 ) ) ;
#7026=CARTESIAN_POINT ( 'NONE',  ( -7.424621202458789426, 7.424621202458724589, 6.000000000000005329 ) ) ;
#7028=FILL_AREA_STYLE_COLOUR ( '', #2926 ) ;
#7032=CARTESIAN_POINT ( 'NONE',  ( -1.642561882922479732, 10.37072757624896191, 6.299999999999972289 ) ) ;
#7035=CARTESIAN_POINT ( 'NONE',  ( -9.377220287598998283, -4.724406229267462898, 1.401137918078568134 ) ) ;
#7036=CARTESIAN_POINT ( 'NONE',  ( -1.612135949262737844, -9.858066664633888365, 6.951137918078597266 ) ) ;
#7047=CARTESIAN_POINT ( 'NONE',  ( -8.900167166472156666, 4.534861676072234893, 17.85000000000001918 ) ) ;
#7048=CARTESIAN_POINT ( 'NONE',  ( 9.865911304835474738, 1.562606840307950051, 1.049999999999966738 ) ) ;
#7058=CARTESIAN_POINT ( 'NONE',  ( 1.689666864740335894, -10.36326688006720786, 8.798862081921429379 ) ) ;
#7063=CARTESIAN_POINT ( 'NONE',  ( 9.383039235653818366, -1.486127417882131097, 13.19999999999998863 ) ) ;
#7064=CARTESIAN_POINT ( 'NONE',  ( 7.806708723663831506, 7.806708723663931870, 18.74999999999998934 ) ) ;
#7069=PLANE ( 'NONE',  #6293 ) ;
#7074=CARTESIAN_POINT ( 'NONE',  ( 7.806708723663831506, 7.806708723663930982, 6.749999999999960032 ) ) ;
#7080=CARTESIAN_POINT ( 'NONE',  ( -4.766900247265192014, -9.355568503977876205, 5.099999999999993427 ) ) ;
#7084=CARTESIAN_POINT ( 'NONE',  ( 1.776620879821457333, 10.89658364409028124, 5.451137918078557298 ) ) ;
#7085=CARTESIAN_POINT ( 'NONE',  ( -8.877401133907129704, 4.579542530753038854, 16.85113791807854611 ) ) ;
#7096=CARTESIAN_POINT ( 'NONE',  ( -8.464561979789474222, -4.312909747525729642, 14.39999999999996838 ) ) ;
#7097=CARTESIAN_POINT ( 'NONE',  ( -9.865911304835474738, -1.562606840307925626, 8.549999999999963407 ) ) ;
#7118=CARTESIAN_POINT ( 'NONE',  ( -1.677562661911643938, -10.91227292449344688, 11.94886208192145993 ) ) ;
#7124=CARTESIAN_POINT ( 'NONE',  ( -8.464561979789474222, -4.312909747525729642, 8.399999999999963052 ) ) ;
#7125=CARTESIAN_POINT ( 'NONE',  ( -7.771249796623103556, -7.842167650704637616, 3.248862081921429112 ) ) ;
#7133=CARTESIAN_POINT ( 'NONE',  ( 1.642561882922480621, -10.37072757624892638, 1.800000000000023803 ) ) ;
#7134=CARTESIAN_POINT ( 'NONE',  ( 9.355568503977840678, 4.766900247265305701, 0.9000000000000119016 ) ) ;
#7138=CARTESIAN_POINT ( 'NONE',  ( -7.806708723663831506, -7.806708723663902560, 17.25000000000003197 ) ) ;
#7142=CARTESIAN_POINT ( 'NONE',  ( 1.776620879821457333, 10.89658364409028124, 8.451137918078549305 ) ) ;
#7143=CARTESIAN_POINT ( 'NONE',  ( 4.355403765523470305, 8.442910196168364578, 11.60113791807856742 ) ) ;
#7154=CARTESIAN_POINT ( 'NONE',  ( -1.562606840307830591, -9.865911304835478290, 16.94999999999998863 ) ) ;
#7155=CARTESIAN_POINT ( 'NONE',  ( 9.383039235653818366, -1.486127417882129986, 7.199999999999984190 ) ) ;
#7164=CARTESIAN_POINT ( 'NONE',  ( -6.751237864895158758, 6.683790977649260334, 0.9988620819214170110 ) ) ;
#7166=CARTESIAN_POINT ( 'NONE',  ( 10.37818827243067510, -1.595456901104499448, 14.19886208192146171 ) ) ;
#7173=CARTESIAN_POINT ( 'NONE',  ( -9.383039235653820143, 1.486127417882155299, 17.69999999999999218 ) ) ;
#7174=CARTESIAN_POINT ( 'NONE',  ( -5.012215536711506658, 9.837026868206022456, 18.15000000000000924 ) ) ;
#7184=CARTESIAN_POINT ( 'NONE',  ( -7.424621202458789426, 7.424621202458720148, 3.000000000000002665 ) ) ;
#7188=CARTESIAN_POINT ( 'NONE',  ( 4.766900247265192903, 9.355568503977902850, 15.60000000000000320 ) ) ;
#7191=CARTESIAN_POINT ( 'NONE',  ( 9.377220287599001836, 4.724406229267492208, 2.901137918078569466 ) ) ;
#7192=CARTESIAN_POINT ( 'NONE',  ( 1.439022436064387511, -9.390499931835517344, 12.80113791807860224 ) ) ;
#7202=CARTESIAN_POINT ( 'NONE',  ( -9.383039235653820143, 1.486127417882155299, 17.69999999999999218 ) ) ;
#7203=CARTESIAN_POINT ( 'NONE',  ( 7.063212654743467489, 7.063212654743553642, 9.749999999999982236 ) ) ;
#7204=CARTESIAN_POINT ( 'NONE',  ( 7.071067811865515473, -7.071067811865425767, 19.50000000000001776 ) ) ;
#7214=CARTESIAN_POINT ( 'NONE',  ( -7.771249796623103556, -7.842167650704634063, 15.24886208192144110 ) ) ;
#7223=CARTESIAN_POINT ( 'NONE',  ( -6.717514421272238856, 6.717514421272180236, 15.00000000000001421 ) ) ;
#7224=CARTESIAN_POINT ( 'NONE',  ( 10.89658364409024749, 1.776620879821585897, 11.04886208192144359 ) ) ;
#7230=CARTESIAN_POINT ( 'NONE',  ( 9.355568503977840678, 4.766900247265305701, 12.90000000000002345 ) ) ;
#7231=CARTESIAN_POINT ( 'NONE',  ( 7.424621202458790314, -7.424621202458697944, 7.500000000000007105 ) ) ;
#7237=CARTESIAN_POINT ( 'NONE',  ( 7.806708723663832394, 7.806708723663926541, 9.749999999999982236 ) ) ;
#7241=CARTESIAN_POINT ( 'NONE',  ( -7.390897758835869524, 7.458344646081644491, 17.00113791807859442 ) ) ;
#7242=CARTESIAN_POINT ( 'NONE',  ( -9.873755945037078874, -1.513077731353020594, 16.55113791807855605 ) ) ;
#7250=CARTESIAN_POINT ( 'NONE',  ( 9.375578539472099848, -1.533232399699987702, 0.2011379180785754783 ) ) ;
#7251=CARTESIAN_POINT ( 'NONE',  ( -4.534861676072319270, 8.900167166472122915, 9.150000000000003908 ) ) ;
#7255=CARTESIAN_POINT ( 'NONE',  ( -1.562606840307830591, -9.865911304835481843, 1.949999999999996403 ) ) ;
#7263=CARTESIAN_POINT ( 'NONE',  ( 6.751237864895159646, -6.683790977649239906, 11.49886208192146775 ) ) ;
#7264=CARTESIAN_POINT ( 'NONE',  ( 9.333916720356675967, 4.809394265263123636, 19.89886208192141481 ) ) ;
#7273=CARTESIAN_POINT ( 'NONE',  ( 4.534861676072321046, -8.900167166472098046, 16.64999999999999858 ) ) ;
#7274=CARTESIAN_POINT ( 'NONE',  ( 9.333916720356675967, 4.809394265263126300, 7.898862081921404155 ) ) ;
#7285=CARTESIAN_POINT ( 'NONE',  ( 7.424621202458790314, -7.424621202458697944, 7.500000000000007105 ) ) ;
#7286=CARTESIAN_POINT ( 'NONE',  ( -7.806708723663830618, -7.806708723663902560, 14.25000000000001243 ) ) ;
#7290=CARTESIAN_POINT ( 'NONE',  ( 1.727091770866551412, 10.90442828429187117, 12.44999999999995666 ) ) ;
#7293=CARTESIAN_POINT ( 'NONE',  ( 10.91227292449344155, 1.677562661911773390, 15.05113791807855961 ) ) ;
#7294=CARTESIAN_POINT ( 'NONE',  ( 7.098671581784200768, 7.027753727702831021, 11.75113791807857666 ) ) ;
#7304=CARTESIAN_POINT ( 'NONE',  ( 6.683790977649321619, -6.751237864895076157, 6.501137918078588207 ) ) ;
#7305=CARTESIAN_POINT ( 'NONE',  ( 9.865911304835474738, 1.562606840307948719, 4.049999999999988276 ) ) ;
#7317=CARTESIAN_POINT ( 'NONE',  ( 1.486127417882244783, -9.383039235653791721, 1.800000000000023803 ) ) ;
#7318=CARTESIAN_POINT ( 'NONE',  ( 9.859792900771104485, -4.967534682030585458, 17.34886208192141765 ) ) ;
#7325=CARTESIAN_POINT ( 'NONE',  ( -8.464561979789474222, -4.312909747525728754, 17.39999999999997016 ) ) ;
#7326=CARTESIAN_POINT ( 'NONE',  ( -1.689666864740335228, 10.36326688006723273, 10.29886208192143293 ) ) ;
#7327=VERTEX_POINT ( 'NONE', #1428 ) ;
#7334=CARTESIAN_POINT ( 'NONE',  ( 5.012215536711511987, -9.837026868205997587, 7.649999999999992362 ) ) ;
#7335=CARTESIAN_POINT ( 'NONE',  ( -1.727091770866549414, -10.90442828429184630, 13.95000000000002593 ) ) ;
#7340=CARTESIAN_POINT ( 'NONE',  ( -7.424621202458789426, 7.424621202458723701, 15.00000000000001421 ) ) ;
#7343=CARTESIAN_POINT ( 'NONE',  ( -10.36326688006724162, 1.689666864740236640, 13.70113791807854398 ) ) ;
#7344=CARTESIAN_POINT ( 'NONE',  ( 4.967534682030706250, -9.859792900771036983, 0.6511379180785785703 ) ) ;
#7349=CARTESIAN_POINT ( 'NONE',  ( 7.806708723663831506, 7.806708723663925653, 9.749999999999982236 ) ) ;
#7355=CARTESIAN_POINT ( 'NONE',  ( -6.683790977649319842, 6.751237864895094809, 2.001137918078543354 ) ) ;
#7356=CARTESIAN_POINT ( 'NONE',  ( -9.865911304835474738, -1.562606840307925626, 14.55000000000000249 ) ) ;
#7366=CARTESIAN_POINT ( 'NONE',  ( 8.922933199037192509, -4.490180821391404287, 17.34886208192141765 ) ) ;
#7367=CARTESIAN_POINT ( 'NONE',  ( -10.89658364409024749, -1.776620879821559917, 18.54886208192142405 ) ) ;
#7373=CARTESIAN_POINT ( 'NONE',  ( 9.865911304835478290, 1.562606840307950273, 19.04999999999997939 ) ) ;
#7374=CARTESIAN_POINT ( 'NONE',  ( 9.859792900771104485, -4.967534682030585458, 8.348862081921442524 ) ) ;
#7381=CARTESIAN_POINT ( 'NONE',  ( 7.806708723663831506, 7.806708723663931870, 3.749999999999997335 ) ) ;
#7389=CARTESIAN_POINT ( 'NONE',  ( 7.806708723663831506, 7.806708723663930982, 0.7499999999999762412 ) ) ;
#7390=CARTESIAN_POINT ( 'NONE',  ( -1.595456901104623348, 10.37818827243067155, 8.301137918078554279 ) ) ;
#7397=CARTESIAN_POINT ( 'NONE',  ( -9.837026868206066865, 5.012215536711416064, 11.84999999999997478 ) ) ;
#7403=CARTESIAN_POINT ( 'NONE',  ( -8.486213763410637156, -4.270415729527909043, 7.401137918078573463 ) ) ;
#7404=CARTESIAN_POINT ( 'NONE',  ( 1.562606840307832368, 9.865911304835510265, 15.44999999999997797 ) ) ;
#7414=CARTESIAN_POINT ( 'NONE',  ( 1.533232399700100945, -9.375578539472067874, 14.79886208192143471 ) ) ;
#7415=CARTESIAN_POINT ( 'NONE',  ( 9.858066664633883036, 1.612135949262857526, 5.048862081921459577 ) ) ;
#7419=DIRECTION ( 'NONE',  ( 1.000000000000000000, 0.000000000000000000, 0.000000000000000000 ) ) ;
#7425=CARTESIAN_POINT ( 'NONE',  ( -1.677562661911643938, -10.91227292449344688, 5.948862081921430622 ) ) ;
#7432=CARTESIAN_POINT ( 'NONE',  ( -7.806708723663830618, -7.806708723663901672, 11.24999999999999467 ) ) ;
#7438=CARTESIAN_POINT ( 'NONE',  ( 10.90442828429184274, 1.727091770866679310, 19.04999999999997939 ) ) ;
#7441=CARTESIAN_POINT ( 'NONE',  ( -1.513077731352923339, -9.873755945037078874, 2.948862081921438616 ) ) ;
#7443=CARTESIAN_POINT ( 'NONE',  ( 7.842167650704563897, 7.771249796623195039, 14.75113791807856956 ) ) ;
#7444=CARTESIAN_POINT ( 'NONE',  ( 9.377220287599001836, 4.724406229267489543, -0.09886208192143307316 ) ) ;
#7449=CARTESIAN_POINT ( 'NONE',  ( -5.012215536711506658, 9.837026868206027785, 12.14999999999996305 ) ) ;
#7455=CARTESIAN_POINT ( 'NONE',  ( 8.877401133907127928, -4.579542530753020202, 6.351137918078572753 ) ) ;
#7456=CARTESIAN_POINT ( 'NONE',  ( 9.383039235653818366, -1.486127417882131097, 16.19999999999999218 ) ) ;
#7468=CARTESIAN_POINT ( 'NONE',  ( 9.858066664633883036, 1.612135949262858858, 14.04886208192143471 ) ) ;
#7469=CARTESIAN_POINT ( 'NONE',  ( 8.922933199037192509, -4.490180821391404287, 8.348862081921442524 ) ) ;
#7483=CARTESIAN_POINT ( 'NONE',  ( 7.424621202458790314, -7.424621202458697944, 19.50000000000001776 ) ) ;
#7492=CARTESIAN_POINT ( 'NONE',  ( -8.922933199037192509, 4.490180821391428267, 3.848862081921410105 ) ) ;
#7494=CARTESIAN_POINT ( 'NONE',  ( -9.355568503977838901, -4.766900247265280832, 2.400000000000013234 ) ) ;
#7495=CARTESIAN_POINT ( 'NONE',  ( 9.814260835641038128, -5.056896391392198709, 3.351137918078579858 ) ) ;
#7500=CARTESIAN_POINT ( 'NONE',  ( -9.355568503977838901, -4.766900247265280832, 8.399999999999963052 ) ) ;
#7506=CARTESIAN_POINT ( 'NONE',  ( 9.375578539472099848, -1.533232399699987702, 12.20113791807854398 ) ) ;
#7507=CARTESIAN_POINT ( 'NONE',  ( -6.717514421272238856, 6.717514421272181124, 18.00000000000001421 ) ) ;
#7520=CARTESIAN_POINT ( 'NONE',  ( -7.027753727702738651, -7.098671581784262941, 15.24886208192144110 ) ) ;
#7521=CARTESIAN_POINT ( 'NONE',  ( 7.027753727702739539, 7.098671581784282480, 4.748862081921425116 ) ) ;
#7523=CARTESIAN_POINT ( 'NONE',  ( -7.424621202458789426, 7.424621202458723701, 15.00000000000001421 ) ) ;
#7535=CARTESIAN_POINT ( 'NONE',  ( 1.727091770866550968, 10.90442828429186761, 18.44999999999999218 ) ) ;
#7543=CARTESIAN_POINT ( 'NONE',  ( -4.270415729527831772, -8.486213763410678013, 3.098862081921434974 ) ) ;
#7544=CARTESIAN_POINT ( 'NONE',  ( -1.727091770866549414, -10.90442828429184274, 7.950000000000040146 ) ) ;
#7545=CARTESIAN_POINT ( 'NONE',  ( 4.809394265263009061, 9.333916720356739916, 5.601137918078562983 ) ) ;
#7548=ADVANCED_FACE ( 'NONE', ( #7684 ), #1122, .T. ) ;
#7549=CARTESIAN_POINT ( 'NONE',  ( 7.806708723663831506, 7.806708723663931870, 3.749999999999997335 ) ) ;
#7556=CARTESIAN_POINT ( 'NONE',  ( 9.375578539472099848, -1.533232399699987702, 15.20113791807854575 ) ) ;
#7557=CARTESIAN_POINT ( 'NONE',  ( 4.534861676072320158, -8.900167166472098046, 13.65000000000003233 ) ) ;
#7570=CARTESIAN_POINT ( 'NONE',  ( -4.766900247265192014, -9.355568503977876205, 2.099999999999990763 ) ) ;
#7571=CARTESIAN_POINT ( 'NONE',  ( -6.717514421272238856, 6.717514421272176683, 3.000000000000002665 ) ) ;
#7572=CARTESIAN_POINT ( 'NONE',  ( -4.270415729527831772, -8.486213763410678013, 12.09886208192144252 ) ) ;
#7573=CARTESIAN_POINT ( 'NONE',  ( -1.727091770866549414, -10.90442828429184630, 16.94999999999998863 ) ) ;
#7581=CARTESIAN_POINT ( 'NONE',  ( 9.355568503977840678, 4.766900247265305701, 12.90000000000002345 ) ) ;
#7585=CARTESIAN_POINT ( 'NONE',  ( -1.642561882922479732, 10.37072757624895303, 15.29999999999997939 ) ) ;
#7593=CARTESIAN_POINT ( 'NONE',  ( 7.424621202458790314, -7.424621202458697944, 19.50000000000001776 ) ) ;
#7596=CARTESIAN_POINT ( 'NONE',  ( 1.513077731352925115, 9.873755945037098414, 4.448862081921434175 ) ) ;
#7598=CARTESIAN_POINT ( 'NONE',  ( -7.806708723663830618, -7.806708723663906113, 8.250000000000028422 ) ) ;
#7599=CARTESIAN_POINT ( 'NONE',  ( 4.967534682030706250, -9.859792900771036983, 15.65113791807858235 ) ) ;
#7607=CARTESIAN_POINT ( 'NONE',  ( 10.90442828429183919, 1.727091770866679532, 13.04999999999999538 ) ) ;
#7613=CARTESIAN_POINT ( 'NONE',  ( 8.486213763410640709, 4.270415729527941018, 11.90113791807857702 ) ) ;
#7614=CARTESIAN_POINT ( 'NONE',  ( -9.873755945037078874, -1.513077731353020594, 7.551137918078578259 ) ) ;
#7626=CARTESIAN_POINT ( 'NONE',  ( -1.642561882922479732, 10.37072757624895303, 0.2999999999999669598 ) ) ;
#7628=CARTESIAN_POINT ( 'NONE',  ( 7.063212654743467489, 7.063212654743553642, 9.749999999999982236 ) ) ;
#7629=CARTESIAN_POINT ( 'NONE',  ( -1.533232399700100057, 9.375578539472089190, 4.298862081921427603 ) ) ;
#7630=CARTESIAN_POINT ( 'NONE',  ( 7.806708723663831506, 7.806708723663925653, 15.74999999999996803 ) ) ;
#7639=CARTESIAN_POINT ( 'NONE',  ( 10.37072757624895836, -1.642561882922355831, 19.19999999999999574 ) ) ;
#7643=CARTESIAN_POINT ( 'NONE',  ( -5.012215536711506658, 9.837026868206022456, 18.15000000000000924 ) ) ;
#7656=CARTESIAN_POINT ( 'NONE',  ( -6.751237864895158758, 6.683790977649260334, 0.9988620819214170110 ) ) ;
#7659=CARTESIAN_POINT ( 'NONE',  ( 7.806708723663831506, 7.806708723663930982, 6.749999999999960032 ) ) ;
#7660=CARTESIAN_POINT ( 'NONE',  ( -1.595456901104623348, 10.37818827243067155, 17.30113791807856316 ) ) ;
#7665=CARTESIAN_POINT ( 'NONE',  ( 10.37072757624895836, -1.642561882922356498, 16.19999999999999218 ) ) ;
#7667=CARTESIAN_POINT ( 'NONE',  ( 4.766900247265192903, 9.355568503977902850, 0.5999999999999894307 ) ) ;
#7672=CARTESIAN_POINT ( 'NONE',  ( 7.842167650704563897, 7.771249796623202144, -0.2488620819214366897 ) ) ;
#7673=CARTESIAN_POINT ( 'NONE',  ( -8.877401133907129704, 4.579542530753042406, 7.851137918078569200 ) ) ;
#7684=FACE_OUTER_BOUND ( 'NONE', #5052, .T. ) ;
#7685=CARTESIAN_POINT ( 'NONE',  ( 4.312909747525650594, 8.464561979789541724, 9.599999999999997868 ) ) ;
#7686=CARTESIAN_POINT ( 'NONE',  ( -9.858066664633883036, -1.612135949262833323, 15.54886208192143293 ) ) ;
#7694=CARTESIAN_POINT ( 'NONE',  ( -7.806708723663830618, -7.806708723663902560, 14.25000000000001243 ) ) ;
#7698=CARTESIAN_POINT ( 'NONE',  ( -1.689666864740335228, 10.36326688006723273, 10.29886208192143293 ) ) ;
#7708=CARTESIAN_POINT ( 'NONE',  ( 4.579542530753127672, -8.877401133907065756, 8.648862081921430800 ) ) ;
#7710=CARTESIAN_POINT ( 'NONE',  ( -7.424621202458789426, 7.424621202458720148, 3.000000000000002665 ) ) ;
#7711=CARTESIAN_POINT ( 'NONE',  ( 10.36326688006723984, -1.689666864740212215, 12.20113791807854398 ) ) ;
#7717=CARTESIAN_POINT ( 'NONE',  ( 10.90442828429184274, 1.727091770866678422, 4.049999999999988276 ) ) ;
#7722=CARTESIAN_POINT ( 'NONE',  ( 8.877401133907127928, -4.579542530753017537, 12.35113791807855677 ) ) ;
#7723=CARTESIAN_POINT ( 'NONE',  ( 6.683790977649321619, -6.751237864895076157, 9.501137918078587319 ) ) ;
#7735=CARTESIAN_POINT ( 'NONE',  ( -7.424621202458789426, 7.424621202458724589, 0.000000000000000000 ) ) ;
#7736=CARTESIAN_POINT ( 'NONE',  ( 8.464561979789474222, 4.312909747525755400, 9.900000000000019895 ) ) ;
#7737=CARTESIAN_POINT ( 'NONE',  ( 1.513077731352925115, 9.873755945037103743, 19.44886208192144039 ) ) ;
#7738=CARTESIAN_POINT ( 'NONE',  ( 7.424621202458790314, -7.424621202458697944, 19.50000000000001776 ) ) ;
#7744=CARTESIAN_POINT ( 'NONE',  ( -5.012215536711506658, 9.837026868206027785, 15.14999999999998259 ) ) ;
#7747=CARTESIAN_POINT ( 'NONE',  ( 7.458344646081711105, -7.390897758835786036, 11.49886208192146775 ) ) ;
#7751=CARTESIAN_POINT ( 'NONE',  ( 6.717514421272239744, -6.717514421272154479, 7.500000000000007105 ) ) ;
#7759=CARTESIAN_POINT ( 'NONE',  ( 10.91227292449344155, 1.677562661911773390, 12.05113791807856671 ) ) ;
#7762=EDGE_CURVE ( 'NONE', #7327, #1139, #4302, .T. ) ;
#7766=CARTESIAN_POINT ( 'NONE',  ( 1.727091770866551412, 10.90442828429186761, 6.449999999999970868 ) ) ;
#7770=CARTESIAN_POINT ( 'NONE',  ( 7.390897758835871301, -7.458344646081617846, 6.501137918078588207 ) ) ;
#7771=CARTESIAN_POINT ( 'NONE',  ( 8.486213763410640709, 4.270415729527937465, 5.901137918078571687 ) ) ;
#7786=CARTESIAN_POINT ( 'NONE',  ( 9.383039235653818366, -1.486127417882129986, 7.199999999999984190 ) ) ;
#7787=CARTESIAN_POINT ( 'NONE',  ( -6.751237864895158758, 6.683790977649255005, 12.99886208192142512 ) ) ;
#7796=CARTESIAN_POINT ( 'NONE',  ( -10.37072757624895836, 1.642561882922380034, 11.69999999999998863 ) ) ;
#7799=CARTESIAN_POINT ( 'NONE',  ( 5.056896391392317724, -9.814260835640970626, 5.648862081921440570 ) ) ;
#7803=CARTESIAN_POINT ( 'NONE',  ( 4.312909747525650594, 8.464561979789541724, 6.599999999999994316 ) ) ;
#7810=CARTESIAN_POINT ( 'NONE',  ( -1.595456901104623348, 10.37818827243067155, 14.30113791807856316 ) ) ;
#7814=CARTESIAN_POINT ( 'NONE',  ( -4.766900247265192014, -9.355568503977867323, 8.099999999999996092 ) ) ;
#7817=CARTESIAN_POINT ( 'NONE',  ( 4.967534682030706250, -9.859792900771036983, 6.651137918078563693 ) ) ;
#7818=CARTESIAN_POINT ( 'NONE',  ( -8.877401133907129704, 4.579542530753039742, 1.851137918078540334 ) ) ;
#7828=CARTESIAN_POINT ( 'NONE',  ( 9.865911304835474738, 1.562606840307950051, 16.04999999999995808 ) ) ;
#7829=CARTESIAN_POINT ( 'NONE',  ( 6.751237864895159646, -6.683790977649233689, 14.49886208192142867 ) ) ;
#7839=CARTESIAN_POINT ( 'NONE',  ( 9.859792900771104485, -4.967534682030585458, 8.348862081921442524 ) ) ;
#7845=CARTESIAN_POINT ( 'NONE',  ( 7.063212654743468377, 7.063212654743558083, 12.75000000000000355 ) ) ;
#7846=CARTESIAN_POINT ( 'NONE',  ( -9.837026868206066865, 5.012215536711416064, 17.85000000000001918 ) ) ;
#7856=CARTESIAN_POINT ( 'NONE',  ( 1.642561882922480621, -10.37072757624892638, 4.800000000000026468 ) ) ;
#7861=CARTESIAN_POINT ( 'NONE',  ( 10.37072757624895836, -1.642561882922355831, 1.200000000000034373 ) ) ;
#7863=CARTESIAN_POINT ( 'NONE',  ( 10.36326688006723984, -1.689666864740212215, 3.201137918078536426 ) ) ;
#7864=CARTESIAN_POINT ( 'NONE',  ( -7.390897758835869524, 7.458344646081644491, -0.9988620819214586444 ) ) ;
#7875=CARTESIAN_POINT ( 'NONE',  ( 4.312909747525650594, 8.464561979789532842, 12.59999999999999964 ) ) ;
#7876=CARTESIAN_POINT ( 'NONE',  ( -4.534861676072319270, 8.900167166472117586, 6.149999999999980815 ) ) ;
#7880=CARTESIAN_POINT ( 'NONE',  ( 8.900167166472158442, -4.534861676072210912, 1.350000000000015410 ) ) ;
#7889=CARTESIAN_POINT ( 'NONE',  ( -9.333916720356675967, -4.809394265263096990, 9.398862081921446787 ) ) ;
#7894=CARTESIAN_POINT ( 'NONE',  ( 4.312909747525650594, 8.464561979789541724, 9.599999999999997868 ) ) ;
#7895=CARTESIAN_POINT ( 'NONE',  ( 7.424621202458790314, -7.424621202458697944, 16.50000000000001421 ) ) ;
#7903=CARTESIAN_POINT ( 'NONE',  ( 7.806708723663831506, 7.806708723663930982, 0.7499999999999762412 ) ) ;
#7904=CARTESIAN_POINT ( 'NONE',  ( 4.766900247265192903, 9.355568503977902850, 3.599999999999992095 ) ) ;
#7906=SURFACE_SIDE_STYLE ('',( #6294 ) ) ;
#7909=CARTESIAN_POINT ( 'NONE',  ( 7.424621202458790314, -7.424621202458697944, 10.50000000000000888 ) ) ;
#7912=CARTESIAN_POINT ( 'NONE',  ( 7.842167650704563897, 7.771249796623202144, 2.751137918078555789 ) ) ;
#7913=CARTESIAN_POINT ( 'NONE',  ( -6.683790977649319842, 6.751237864895094809, 11.00113791807855002 ) ) ;
#7925=CARTESIAN_POINT ( 'NONE',  ( -8.464561979789474222, -4.312909747525728754, 17.39999999999997016 ) ) ;
#7926=CARTESIAN_POINT ( 'NONE',  ( 6.717514421272239744, -6.717514421272154479, 7.500000000000007105 ) ) ;
#7930=CARTESIAN_POINT ( 'NONE',  ( 9.383039235653818366, -1.486127417882129986, 4.199999999999981526 ) ) ;
#7937=CARTESIAN_POINT ( 'NONE',  ( -7.424621202458789426, 7.424621202458724589, -3.058133128536869244E-17 ) ) ;
#7939=CARTESIAN_POINT ( 'NONE',  ( -1.677562661911643938, -10.91227292449344688, 17.94886208192144395 ) ) ;
#7942=CARTESIAN_POINT ( 'NONE',  ( -10.89658364409024749, -1.776620879821561694, 15.54886208192143293 ) ) ;
#7949=CARTESIAN_POINT ( 'NONE',  ( 1.486127417882244783, -9.383039235653782839, 10.80000000000003268 ) ) ;
#7951=CARTESIAN_POINT ( 'NONE',  ( -5.012215536711506658, 9.837026868206027785, 15.14999999999998259 ) ) ;
#7957=DIRECTION ( 'NONE',  ( 0.7063021515967560227, 0.7063021515967630171, 0.04769215134145720486 ) ) ;
#7958=CARTESIAN_POINT ( 'NONE',  ( -9.355568503977838901, -4.766900247265279944, 5.400000000000016342 ) ) ;
#7963=CARTESIAN_POINT ( 'NONE',  ( 7.424621202458790314, -7.424621202458697944, 13.50000000000001243 ) ) ;
#7967=CARTESIAN_POINT ( 'NONE',  ( -9.377220287598998283, -4.724406229267462898, 4.401137918078569022 ) ) ;
#7968=CARTESIAN_POINT ( 'NONE',  ( -9.375578539472099848, 1.533232399700011461, 13.70113791807854398 ) ) ;
#7980=CARTESIAN_POINT ( 'NONE',  ( -7.063212654743466601, -7.063212654743531438, 14.25000000000001243 ) ) ;
#7981=CARTESIAN_POINT ( 'NONE',  ( 9.383039235653818366, -1.486127417882129986, 10.19999999999998685 ) ) ;
#7984=CARTESIAN_POINT ( 'NONE',  ( -1.486127417882243895, 9.383039235653816590, 3.299999999999969624 ) ) ;
#7991=CARTESIAN_POINT ( 'NONE',  ( -7.027753727702738651, -7.098671581784262941, 9.248862081921457090 ) ) ;
#7992=CARTESIAN_POINT ( 'NONE',  ( -9.859792900771106261, 4.967534682030607662, 15.84886208192146739 ) ) ;
#7999=CARTESIAN_POINT ( 'NONE',  ( -9.859792900771106261, 4.967534682030611215, 9.848862081921437195 ) ) ;
#8005=CARTESIAN_POINT ( 'NONE',  ( -1.642561882922479732, 10.37072757624895303, 12.29999999999997762 ) ) ;
#8006=CARTESIAN_POINT ( 'NONE',  ( 10.90442828429183919, 1.727091770866679310, 7.050000000000010481 ) ) ;
#8010=CARTESIAN_POINT ( 'NONE',  ( -9.837026868206070418, 5.012215536711416952, 17.85000000000001918 ) ) ;
#8014=CARTESIAN_POINT ( 'NONE',  ( 1.776620879821457333, 10.89658364409028124, 11.45113791807854220 ) ) ;
#8015=CARTESIAN_POINT ( 'NONE',  ( 1.439022436064387511, -9.390499931835510239, 15.80113791807855961 ) ) ;
#8025=CARTESIAN_POINT ( 'NONE',  ( -8.900167166472156666, 4.534861676072231340, 14.84999999999999787 ) ) ;
#8026=CARTESIAN_POINT ( 'NONE',  ( 4.534861676072320158, -8.900167166472098046, 10.65000000000000924 ) ) ;
#8030=CARTESIAN_POINT ( 'NONE',  ( -4.534861676072319270, 8.900167166472122915, 0.1499999999999952482 ) ) ;
#8032=EDGE_CURVE ( 'NONE', #8995, #879, #9592, .T. ) ;
#8039=CARTESIAN_POINT ( 'NONE',  ( 9.858066664633883036, 1.612135949262857082, 8.048862081921450695 ) ) ;
#8040=CARTESIAN_POINT ( 'NONE',  ( -10.37818827243067688, 1.595456901104524761, 18.69886208192145816 ) ) ;
#8048=CARTESIAN_POINT ( 'NONE',  ( -7.771249796623103556, -7.842167650704634063, 6.248862081921465084 ) ) ;
#8054=CARTESIAN_POINT ( 'NONE',  ( -7.806708723663830618, -7.806708723663901672, 5.250000000000008882 ) ) ;
#8055=CARTESIAN_POINT ( 'NONE',  ( 9.837026868206066865, -5.012215536711392083, 13.34999999999998188 ) ) ;
#8061=CARTESIAN_POINT ( 'NONE',  ( 9.837026868206070418, -5.012215536711391195, 10.35000000000002274 ) ) ;
#8065=CARTESIAN_POINT ( 'NONE',  ( -7.842167650704559456, -7.771249796623176387, 16.25113791807856245 ) ) ;
#8066=CARTESIAN_POINT ( 'NONE',  ( 8.877401133907127928, -4.579542530753017537, 12.35113791807855677 ) ) ;
#8076=CARTESIAN_POINT ( 'NONE',  ( 7.424621202458790314, -7.424621202458697944, 19.50000000000001776 ) ) ;
#8077=CARTESIAN_POINT ( 'NONE',  ( 1.439022436064387511, -9.390499931835510239, 6.801137918078597799 ) ) ;
#8078=CARTESIAN_POINT ( 'NONE',  ( -1.562606840307830591, -9.865911304835476514, 7.950000000000040146 ) ) ;
#8083=CIRCLE ( 'NONE', #1323, 0.4999999999999994449 ) ;
#8087=SURFACE_SIDE_STYLE ('',( #1788 ) ) ;
#8090=CARTESIAN_POINT ( 'NONE',  ( 8.900167166472154889, -4.534861676072210912, 1.350000000000015188 ) ) ;
#8091=CARTESIAN_POINT ( 'NONE',  ( 7.458344646081711105, -7.390897758835786036, 20.49886208192143400 ) ) ;
#8101=CARTESIAN_POINT ( 'NONE',  ( -7.063212654743467489, -7.063212654743533214, 17.25000000000003197 ) ) ;
#8102=CARTESIAN_POINT ( 'NONE',  ( 7.458344646081711105, -7.390897758835778930, 5.498862081921462419 ) ) ;
#8111=CARTESIAN_POINT ( 'NONE',  ( -4.766900247265192014, -9.355568503977876205, 5.099999999999993427 ) ) ;
#8112=CARTESIAN_POINT ( 'NONE',  ( 1.727091770866550968, 10.90442828429186761, 18.44999999999999218 ) ) ;
#8116=CARTESIAN_POINT ( 'NONE',  ( -1.642561882922479732, 10.37072757624896191, 9.299999999999975842 ) ) ;
#8120=CARTESIAN_POINT ( 'NONE',  ( 10.91227292449344155, 1.677562661911773167, 18.05113791807859513 ) ) ;
#8121=CARTESIAN_POINT ( 'NONE',  ( -10.36326688006724162, 1.689666864740236640, 1.701137918078535094 ) ) ;
#8128=CARTESIAN_POINT ( 'NONE',  ( -4.355403765523468529, -8.442910196168346815, 10.10113791807856742 ) ) ;
#8129=CARTESIAN_POINT ( 'NONE',  ( -8.900167166472156666, 4.534861676072234893, 11.84999999999997478 ) ) ;
#8138=CARTESIAN_POINT ( 'NONE',  ( 4.270415729527831772, 8.486213763410697553, 16.59886208192144252 ) ) ;
#8140=CARTESIAN_POINT ( 'NONE',  ( -9.859792900771106261, 4.967534682030611215, 18.84886208192146029 ) ) ;
#8147=CARTESIAN_POINT ( 'NONE',  ( 7.063212654743468377, 7.063212654743554531, 15.74999999999996803 ) ) ;
#8148=CARTESIAN_POINT ( 'NONE',  ( 10.89658364409024749, 1.776620879821585897, 5.048862081921459577 ) ) ;
#8155=CARTESIAN_POINT ( 'NONE',  ( 10.90442828429183919, 1.727091770866679310, 7.050000000000010481 ) ) ;
#8162=CARTESIAN_POINT ( 'NONE',  ( 10.36326688006723984, -1.689666864740212215, 15.20113791807854575 ) ) ;
#8163=CARTESIAN_POINT ( 'NONE',  ( 9.814260835641038128, -5.056896391392198709, 0.3511379180785880183 ) ) ;
#8167=CARTESIAN_POINT ( 'NONE',  ( -1.727091770866549414, -10.90442828429184274, 7.950000000000040146 ) ) ;
#8176=CARTESIAN_POINT ( 'NONE',  ( -4.355403765523468529, -8.442910196168346815, 1.101137918078559208 ) ) ;
#8177=CARTESIAN_POINT ( 'NONE',  ( 1.612135949262739398, 9.858066664633913234, -0.5488620819214271584 ) ) ;
#8188=CARTESIAN_POINT ( 'NONE',  ( -8.922933199037192509, 4.490180821391425603, 15.84886208192146739 ) ) ;
#8189=CARTESIAN_POINT ( 'NONE',  ( -9.390499931835536884, 1.439022436064298249, 9.698862081921454603 ) ) ;
#8196=CARTESIAN_POINT ( 'NONE',  ( -1.677562661911643938, -10.91227292449344688, 8.948862081921467038 ) ) ;
#8203=CARTESIAN_POINT ( 'NONE',  ( 7.424621202458790314, -7.424621202458697944, 10.50000000000000888 ) ) ;
#8212=CARTESIAN_POINT ( 'NONE',  ( -9.814260835641038128, 5.056896391392219137, 10.85113791807856209 ) ) ;
#8213=CARTESIAN_POINT ( 'NONE',  ( 1.776620879821457333, 10.89658364409028124, 2.451137918078564848 ) ) ;
#8220=CARTESIAN_POINT ( 'NONE',  ( 7.424621202458790314, -7.424621202458697944, 10.50000000000000888 ) ) ;
#8226=CARTESIAN_POINT ( 'NONE',  ( 9.375578539472099848, -1.533232399699986370, 6.201137918078538647 ) ) ;
#8227=CARTESIAN_POINT ( 'NONE',  ( 8.464561979789474222, 4.312909747525755400, 15.90000000000002522 ) ) ;
#8238=CARTESIAN_POINT ( 'NONE',  ( -8.442910196168309511, -4.355403765523546689, 15.39886208192141126 ) ) ;
#8239=CARTESIAN_POINT ( 'NONE',  ( 9.390499931835536884, -1.439022436064272270, 11.19886208192145816 ) ) ;
#8256=CARTESIAN_POINT ( 'NONE',  ( -7.806708723663830618, -7.806708723663901672, 17.25000000000003553 ) ) ;
#8266=CARTESIAN_POINT ( 'NONE',  ( 7.027753727702739539, 7.098671581784282480, 4.748862081921425116 ) ) ;
#8268=CARTESIAN_POINT ( 'NONE',  ( -5.012215536711506658, 9.837026868206027785, 3.149999999999957723 ) ) ;
#8269=CARTESIAN_POINT ( 'NONE',  ( -9.814260835641038128, 5.056896391392221801, 4.851137918078532785 ) ) ;
#8275=CARTESIAN_POINT ( 'NONE',  ( -10.90442828429183919, -1.727091770866655329, 5.549999999999999822 ) ) ;
#8281=CARTESIAN_POINT ( 'NONE',  ( -9.375578539472099848, 1.533232399700010351, 7.701137918078540423 ) ) ;
#8282=CARTESIAN_POINT ( 'NONE',  ( -8.900167166472156666, 4.534861676072234893, 17.85000000000001918 ) ) ;
#8296=CARTESIAN_POINT ( 'NONE',  ( 9.390499931835536884, -1.439022436064273158, 20.19886208192146526 ) ) ;
#8297=CARTESIAN_POINT ( 'NONE',  ( -6.751237864895158758, 6.683790977649261222, 6.998862081921422451 ) ) ;
#8298=CARTESIAN_POINT ( 'NONE',  ( -5.012215536711506658, 9.837026868206027785, 12.14999999999996305 ) ) ;
#8313=CARTESIAN_POINT ( 'NONE',  ( 9.837026868206066865, -5.012215536711395636, 16.35000000000000497 ) ) ;
#8321=CARTESIAN_POINT ( 'NONE',  ( 7.458344646081711105, -7.390897758835786036, 20.49886208192143400 ) ) ;
#8323=CARTESIAN_POINT ( 'NONE',  ( 1.642561882922480621, -10.37072757624891750, 7.800000000000029132 ) ) ;
#8324=CARTESIAN_POINT ( 'NONE',  ( 1.595456901104624459, -10.37818827243065201, 3.801137918078595135 ) ) ;
#8327=CARTESIAN_POINT ( 'NONE',  ( -7.424621202458789426, 7.424621202458720148, 3.000000000000002665 ) ) ;
#8332=CARTESIAN_POINT ( 'NONE',  ( 6.683790977649321619, -6.751237864895082375, 12.50113791807859265 ) ) ;
#8333=CARTESIAN_POINT ( 'NONE',  ( -6.717514421272238856, 6.717514421272180236, 15.00000000000001421 ) ) ;
#8344=CARTESIAN_POINT ( 'NONE',  ( 9.865911304835474738, 1.562606840307949829, 7.050000000000010481 ) ) ;
#8345=CARTESIAN_POINT ( 'NONE',  ( 4.270415729527831772, 8.486213763410688671, 4.598862081921435419 ) ) ;
#8347=CARTESIAN_POINT ( 'NONE',  ( 10.90442828429183919, 1.727091770866679532, 16.04999999999995808 ) ) ;
#8356=CARTESIAN_POINT ( 'NONE',  ( 7.806708723663831506, 7.806708723663931870, 18.74999999999998934 ) ) ;
#8360=CARTESIAN_POINT ( 'NONE',  ( 1.689666864740335894, -10.36326688006721497, 2.798862081921426714 ) ) ;
#8365=CARTESIAN_POINT ( 'NONE',  ( -1.642561882922479732, 10.37072757624895303, 18.29999999999998295 ) ) ;
#8369=CARTESIAN_POINT ( 'NONE',  ( 6.751237864895159646, -6.683790977649239906, 2.498862081921459755 ) ) ;
#8370=CARTESIAN_POINT ( 'NONE',  ( -5.012215536711506658, 9.837026868206022456, 6.149999999999980815 ) ) ;
#8371=CARTESIAN_POINT ( 'NONE',  ( -1.776620879821455556, -10.89658364409025637, 12.95113791807858128 ) ) ;
#8376=CARTESIAN_POINT ( 'NONE',  ( 7.424621202458790314, -7.424621202458697944, 7.500000000000007105 ) ) ;
#8381=CARTESIAN_POINT ( 'NONE',  ( 9.873755945037075321, 1.513077731353044131, 18.05113791807859513 ) ) ;
#8382=CARTESIAN_POINT ( 'NONE',  ( 1.439022436064387511, -9.390499931835510239, 6.801137918078597799 ) ) ;
#8393=CARTESIAN_POINT ( 'NONE',  ( 8.900167166472154889, -4.534861676072210912, 7.350000000000000533 ) ) ;
#8394=CARTESIAN_POINT ( 'NONE',  ( -4.270415729527831772, -8.486213763410678013, 3.098862081921434974 ) ) ;
#8395=CARTESIAN_POINT ( 'NONE',  ( 10.37072757624895836, -1.642561882922355609, 10.19999999999998685 ) ) ;
#8403=CARTESIAN_POINT ( 'NONE',  ( 10.90442828429183919, 1.727091770866679532, 16.04999999999995808 ) ) ;
#8408=CARTESIAN_POINT ( 'NONE',  ( 4.766900247265192903, 9.355568503977902850, 15.60000000000000320 ) ) ;
#8421=CARTESIAN_POINT ( 'NONE',  ( 7.771249796623105333, 7.842167650704658932, 16.74886208192143755 ) ) ;
#8422=CARTESIAN_POINT ( 'NONE',  ( 10.37072757624895836, -1.642561882922355609, 10.19999999999998685 ) ) ;
#8423=CARTESIAN_POINT ( 'NONE',  ( -7.390897758835869524, 7.458344646081644491, 17.00113791807859442 ) ) ;
#8428=( NAMED_UNIT ( * ) SI_UNIT ( $, .STERADIAN. ) SOLID_ANGLE_UNIT ( ) );
#8429=CARTESIAN_POINT ( 'NONE',  ( -4.724406229267374968, -9.377220287599046245, 3.098862081921434974 ) ) ;
#8431=CARTESIAN_POINT ( 'NONE',  ( 9.837026868206070418, -5.012215536711392083, 1.350000000000015410 ) ) ;
#8438=CARTESIAN_POINT ( 'NONE',  ( 1.776620879821457333, 10.89658364409028124, -0.5488620819214271584 ) ) ;
#8439=CARTESIAN_POINT ( 'NONE',  ( -4.490180821391513533, 8.922933199037158758, 2.151137918078574796 ) ) ;
#8450=CARTESIAN_POINT ( 'NONE',  ( -4.534861676072319270, 8.900167166472121139, 3.149999999999957723 ) ) ;
#8451=CARTESIAN_POINT ( 'NONE',  ( 4.270415729527831772, 8.486213763410697553, 16.59886208192144252 ) ) ;
#8462=CARTESIAN_POINT ( 'NONE',  ( 10.90442828429183919, 1.727091770866679532, 13.04999999999999538 ) ) ;
#8467=CARTESIAN_POINT ( 'NONE',  ( 10.37818827243067510, -1.595456901104499448, 2.198862081921450606 ) ) ;
#8479=CARTESIAN_POINT ( 'NONE',  ( 1.533232399700100945, -9.375578539472073203, 2.798862081921426714 ) ) ;
#8482=CARTESIAN_POINT ( 'NONE',  ( 7.424621202458790314, -7.424621202458697944, 4.500000000000003553 ) ) ;
#8483=CARTESIAN_POINT ( 'NONE',  ( -5.012215536711506658, 9.837026868206027785, 0.1499999999999952482 ) ) ;
#8488=CARTESIAN_POINT ( 'NONE',  ( -5.012215536711508435, 9.837026868206020680, 6.149999999999979927 ) ) ;
#8492=CARTESIAN_POINT ( 'NONE',  ( 6.683790977649321619, -6.751237864895076157, 15.50113791807859620 ) ) ;
#8493=CARTESIAN_POINT ( 'NONE',  ( -9.873755945037078874, -1.513077731353020594, 1.551137918078593803 ) ) ;
#8503=CARTESIAN_POINT ( 'NONE',  ( -1.562606840307830591, -9.865911304835488949, 4.950000000000017053 ) ) ;
#8504=CARTESIAN_POINT ( 'NONE',  ( -6.751237864895158758, 6.683790977649261222, 15.99886208192142512 ) ) ;
#8518=CARTESIAN_POINT ( 'NONE',  ( -10.89658364409024749, -1.776620879821561472, 12.54886208192144004 ) ) ;
#8523=CARTESIAN_POINT ( 'NONE',  ( 8.900167166472158442, -4.534861676072210024, 10.35000000000002274 ) ) ;
#8529=CARTESIAN_POINT ( 'NONE',  ( 7.027753727702739539, 7.098671581784288698, 10.74886208192140913 ) ) ;
#8532=CARTESIAN_POINT ( 'NONE',  ( 7.390897758835871301, -7.458344646081617846, 9.501137918078587319 ) ) ;
#8538=CARTESIAN_POINT ( 'NONE',  ( 1.642561882922480621, -10.37072757624892638, 4.800000000000026468 ) ) ;
#8543=CARTESIAN_POINT ( 'NONE',  ( -8.877401133907129704, 4.579542530753039742, 10.85113791807856209 ) ) ;
#8544=CARTESIAN_POINT ( 'NONE',  ( -1.612135949262737844, -9.858066664633888365, 0.9511379180785689558 ) ) ;
#8554=CARTESIAN_POINT ( 'NONE',  ( -8.900167166472156666, 4.534861676072231340, 8.850000000000008527 ) ) ;
#8555=CARTESIAN_POINT ( 'NONE',  ( -1.533232399700100057, 9.375578539472094519, 19.29886208192143471 ) ) ;
#8556=DIRECTION ( 'NONE',  ( -0.7071067811865510144, 0.7071067811865440200, -6.116266257073745883E-17 ) ) ;
#8562=CARTESIAN_POINT ( 'NONE',  ( 4.766900247265192903, 9.355568503977902850, 12.59999999999999964 ) ) ;
#8567=CARTESIAN_POINT ( 'NONE',  ( 10.37818827243067510, -1.595456901104500780, 5.198862081921453715 ) ) ;
#8572=CARTESIAN_POINT ( 'NONE',  ( -1.486127417882243895, 9.383039235653816590, 12.29999999999997762 ) ) ;
#8579=CARTESIAN_POINT ( 'NONE',  ( -9.390499931835536884, 1.439022436064298249, 9.698862081921454603 ) ) ;
#8581=CARTESIAN_POINT ( 'NONE',  ( -7.424621202458789426, 7.424621202458720148, 3.000000000000002665 ) ) ;
#8582=CARTESIAN_POINT ( 'NONE',  ( -9.377220287598998283, -4.724406229267462898, 16.40113791807857524 ) ) ;
#8589=CARTESIAN_POINT ( 'NONE',  ( 5.012215536711512875, -9.837026868206002916, 7.649999999999992362 ) ) ;
#8592=CARTESIAN_POINT ( 'NONE',  ( 4.967534682030706250, -9.859792900771036983, 9.651137918078598332 ) ) ;
#8593=CARTESIAN_POINT ( 'NONE',  ( 8.486213763410640709, 4.270415729527940130, 2.901137918078569466 ) ) ;
#8608=CARTESIAN_POINT ( 'NONE',  ( 7.098671581784200768, 7.027753727702831021, -0.2488620819214366897 ) ) ;
#8609=CARTESIAN_POINT ( 'NONE',  ( -4.579542530753125895, 8.877401133907083519, 13.14886208192146633 ) ) ;
#8624=CARTESIAN_POINT ( 'NONE',  ( 10.37818827243067510, -1.595456901104500780, 8.198862081921454603 ) ) ;
#8629=CARTESIAN_POINT ( 'NONE',  ( 1.562606840307832146, 9.865911304835508489, 12.44999999999995666 ) ) ;
#8630=CARTESIAN_POINT ( 'NONE',  ( 1.642561882922480621, -10.37072757624892638, 16.80000000000003624 ) ) ;
#8640=CARTESIAN_POINT ( 'NONE',  ( 1.642561882922480621, -10.37072757624892638, 1.800000000000023803 ) ) ;
#8645=CARTESIAN_POINT ( 'NONE',  ( -10.37072757624895836, 1.642561882922380923, 2.699999999999980194 ) ) ;
#8648=CARTESIAN_POINT ( 'NONE',  ( -10.91227292449344155, -1.677562661911747632, 1.551137918078593803 ) ) ;
#8649=CARTESIAN_POINT ( 'NONE',  ( 9.375578539472099848, -1.533232399699986370, 18.20113791807854398 ) ) ;
#8660=CARTESIAN_POINT ( 'NONE',  ( -1.612135949262737844, -9.858066664633888365, 0.9511379180785689558 ) ) ;
#8661=CARTESIAN_POINT ( 'NONE',  ( -9.390499931835536884, 1.439022436064298249, 18.69886208192145816 ) ) ;
#8674=CARTESIAN_POINT ( 'NONE',  ( -4.724406229267374968, -9.377220287599040915, 6.098862081921437195 ) ) ;
#8678=CARTESIAN_POINT ( 'NONE',  ( -4.312909747525649706, -8.464561979789507973, 14.10000000000000142 ) ) ;
#8679=CARTESIAN_POINT ( 'NONE',  ( 10.37818827243067510, -1.595456901104499448, 2.198862081921450606 ) ) ;
#8686=CARTESIAN_POINT ( 'NONE',  ( 7.424621202458790314, -7.424621202458697944, 1.500000000000001332 ) ) ;
#8687=CARTESIAN_POINT ( 'NONE',  ( -10.37072757624895836, 1.642561882922380923, 2.699999999999980194 ) ) ;
#8693=CARTESIAN_POINT ( 'NONE',  ( -9.355568503977838901, -4.766900247265279944, 11.39999999999996660 ) ) ;
#8696=CARTESIAN_POINT ( 'NONE',  ( -10.36326688006724162, 1.689666864740236640, 1.701137918078535094 ) ) ;
#8697=CARTESIAN_POINT ( 'NONE',  ( 6.683790977649321619, -6.751237864895076157, 15.50113791807859620 ) ) ;
#8707=CARTESIAN_POINT ( 'NONE',  ( 9.383039235653818366, -1.486127417882131097, 16.19999999999999218 ) ) ;
#8708=CARTESIAN_POINT ( 'NONE',  ( 4.534861676072320158, -8.900167166472096270, 7.649999999999992362 ) ) ;
#8719=CARTESIAN_POINT ( 'NONE',  ( 4.579542530753127672, -8.877401133907065756, 2.648862081921448119 ) ) ;
#8721=CARTESIAN_POINT ( 'NONE',  ( -4.724406229267374968, -9.377220287599046245, 12.09886208192144252 ) ) ;
#8728=CARTESIAN_POINT ( 'NONE',  ( -1.486127417882243895, 9.383039235653825472, 9.299999999999975842 ) ) ;
#8729=CARTESIAN_POINT ( 'NONE',  ( -7.424621202458789426, 7.424621202458723701, 15.00000000000001421 ) ) ;
#8736=CARTESIAN_POINT ( 'NONE',  ( -10.37072757624895836, 1.642561882922380923, 2.699999999999980194 ) ) ;
#8737=CARTESIAN_POINT ( 'NONE',  ( 1.727091770866550968, 10.90442828429187294, 3.450000000000006839 ) ) ;
#8739=SHAPE_REPRESENTATION_RELATIONSHIP ( 'NONE' , 'NONE' ,  #1843, #9458 ) ;
#8742=CARTESIAN_POINT ( 'NONE',  ( 5.012215536711512875, -9.837026868206002916, 16.64999999999999858 ) ) ;
#8745=CARTESIAN_POINT ( 'NONE',  ( -1.595456901104623348, 10.37818827243066622, 2.301137918078551614 ) ) ;
#8746=CARTESIAN_POINT ( 'NONE',  ( 7.098671581784200768, 7.027753727702823916, 14.75113791807856956 ) ) ;
#8749=MECHANICAL_DESIGN_GEOMETRIC_PRESENTATION_REPRESENTATION('',(#6274),#4284);
#8757=CARTESIAN_POINT ( 'NONE',  ( 4.355403765523470305, 8.442910196168369907, -0.3988620819214416247 ) ) ;
#8758=CARTESIAN_POINT ( 'NONE',  ( 7.063212654743467489, 7.063212654743557195, 6.749999999999960032 ) ) ;
#8761=CARTESIAN_POINT ( 'NONE',  ( 7.063212654743468377, 7.063212654743559860, 3.749999999999997780 ) ) ;
#8774=CARTESIAN_POINT ( 'NONE',  ( -9.858066664633883036, -1.612135949262831547, 6.548862081921412504 ) ) ;
#8775=CARTESIAN_POINT ( 'NONE',  ( 7.458344646081711105, -7.390897758835778930, 14.49886208192142867 ) ) ;
#8779=CARTESIAN_POINT ( 'NONE',  ( -4.724406229267374968, -9.377220287599040915, 15.09886208192144430 ) ) ;
#8785=CARTESIAN_POINT ( 'NONE',  ( -6.717514421272238856, 6.717514421272181124, 18.00000000000001421 ) ) ;
#8787=CARTESIAN_POINT ( 'NONE',  ( 9.355568503977840678, 4.766900247265305701, 12.90000000000002345 ) ) ;
#8793=CARTESIAN_POINT ( 'NONE',  ( -7.424621202458789426, 7.424621202458724589, 12.00000000000001066 ) ) ;
#8794=CARTESIAN_POINT ( 'NONE',  ( 7.424621202458790314, -7.424621202458697944, 1.500000000000001332 ) ) ;
#8800=CARTESIAN_POINT ( 'NONE',  ( 7.424621202458790314, -7.424621202458697944, 16.50000000000001421 ) ) ;
#8805=CARTESIAN_POINT ( 'NONE',  ( -10.91227292449344155, -1.677562661911748965, 7.551137918078578259 ) ) ;
#8806=CARTESIAN_POINT ( 'NONE',  ( -1.439022436064386845, 9.390499931835535108, 14.30113791807856316 ) ) ;
#8818=CARTESIAN_POINT ( 'NONE',  ( 7.063212654743467489, 7.063212654743553642, 15.74999999999996803 ) ) ;
#8819=CARTESIAN_POINT ( 'NONE',  ( 6.717514421272239744, -6.717514421272154479, 10.50000000000000888 ) ) ;
#8830=CARTESIAN_POINT ( 'NONE',  ( -8.442910196168309511, -4.355403765523546689, 9.398862081921404155 ) ) ;
#8831=CARTESIAN_POINT ( 'NONE',  ( 10.37818827243067510, -1.595456901104500780, 17.19886208192146171 ) ) ;
#8838=CARTESIAN_POINT ( 'NONE',  ( -9.333916720356675967, -4.809394265263096990, 6.398862081921446787 ) ) ;
#8847=CARTESIAN_POINT ( 'NONE',  ( 10.37072757624895836, -1.642561882922355609, 4.199999999999981526 ) ) ;
#8848=CARTESIAN_POINT ( 'NONE',  ( -5.012215536711506658, 9.837026868206027785, 3.149999999999957723 ) ) ;
#8852=CARTESIAN_POINT ( 'NONE',  ( -1.642561882922479732, 10.37072757624895303, 12.29999999999997762 ) ) ;
#8855=CARTESIAN_POINT ( 'NONE',  ( 1.595456901104624459, -10.37818827243064490, 15.80113791807855961 ) ) ;
#8856=CARTESIAN_POINT ( 'NONE',  ( -1.439022436064386845, 9.390499931835535108, 17.30113791807856316 ) ) ;
#8864=CARTESIAN_POINT ( 'NONE',  ( 4.355403765523470305, 8.442910196168369907, 8.601137918078563871 ) ) ;
#8865=CARTESIAN_POINT ( 'NONE',  ( -7.063212654743466601, -7.063212654743534991, 8.250000000000028422 ) ) ;
#8875=CARTESIAN_POINT ( 'NONE',  ( 8.442910196168311288, 4.355403765523574222, 13.89886208192141126 ) ) ;
#8877=CARTESIAN_POINT ( 'NONE',  ( 8.442910196168311288, 4.355403765523574222, 1.898862081921442790 ) ) ;
#8883=CARTESIAN_POINT ( 'NONE',  ( 8.464561979789474222, 4.312909747525755400, 15.90000000000002522 ) ) ;
#8884=CARTESIAN_POINT ( 'NONE',  ( -9.859792900771106261, 4.967534682030611215, 12.84886208192143009 ) ) ;
#8892=CARTESIAN_POINT ( 'NONE',  ( 4.766900247265192903, 9.355568503977911732, 9.599999999999997868 ) ) ;
#8893=CARTESIAN_POINT ( 'NONE',  ( -10.90442828429183919, -1.727091770866654663, 17.55000000000002913 ) ) ;
#8897=CARTESIAN_POINT ( 'NONE',  ( -10.90442828429184274, -1.727091770866655107, 11.54999999999998295 ) ) ;
#8900=CARTESIAN_POINT ( 'NONE',  ( 7.390897758835871301, -7.458344646081624063, 12.50113791807859265 ) ) ;
#8901=CARTESIAN_POINT ( 'NONE',  ( 7.842167650704563897, 7.771249796623202144, -0.2488620819214366897 ) ) ;
#8911=CARTESIAN_POINT ( 'NONE',  ( 4.490180821391514421, -8.922933199037132113, 6.651137918078563693 ) ) ;
#8912=CARTESIAN_POINT ( 'NONE',  ( -4.312909747525649706, -8.464561979789499091, 8.099999999999996092 ) ) ;
#8923=CARTESIAN_POINT ( 'NONE',  ( -7.063212654743466601, -7.063212654743534991, 2.249999999999986233 ) ) ;
#8924=CARTESIAN_POINT ( 'NONE',  ( 9.333916720356675967, 4.809394265263126300, 16.89886208192141126 ) ) ;
#8926=AXIS2_PLACEMENT_3D ( 'NONE', #9751, #4211, #6475 ) ;
#8930=DIRECTION ( 'NONE',  ( 0.000000000000000000, 0.000000000000000000, 1.000000000000000000 ) ) ;
#8934=CARTESIAN_POINT ( 'NONE',  ( -8.900167166472160218, 4.534861676072235781, 17.85000000000001918 ) ) ;
#8935=CARTESIAN_POINT ( 'NONE',  ( 9.859792900771104485, -4.967534682030588122, 11.34886208192143364 ) ) ;
#8945=CARTESIAN_POINT ( 'NONE',  ( -4.766900247265192014, -9.355568503977867323, 11.09999999999999787 ) ) ;
#8946=CARTESIAN_POINT ( 'NONE',  ( -10.37072757624895836, 1.642561882922380034, 11.69999999999998863 ) ) ;
#8956=CARTESIAN_POINT ( 'NONE',  ( 1.727091770866550968, 10.90442828429187294, 0.4499999999999856337 ) ) ;
#8957=CARTESIAN_POINT ( 'NONE',  ( -4.967534682030703586, 9.859792900771061852, 5.151137918078567246 ) ) ;
#8963=CARTESIAN_POINT ( 'NONE',  ( 4.766900247265192903, 9.355568503977902850, 3.599999999999992095 ) ) ;
#8971=CARTESIAN_POINT ( 'NONE',  ( 8.877401133907127928, -4.579542530753017537, 3.351137918078579858 ) ) ;
#8972=CARTESIAN_POINT ( 'NONE',  ( 1.562606840307832368, 9.865911304835510265, 12.44999999999995666 ) ) ;
#8983=CARTESIAN_POINT ( 'NONE',  ( 4.270415729527831772, 8.486213763410697553, 7.598862081921438971 ) ) ;
#8990=CARTESIAN_POINT ( 'NONE',  ( 1.486127417882244783, -9.383039235653791721, 16.80000000000003624 ) ) ;
#8991=CARTESIAN_POINT ( 'NONE',  ( 7.458344646081711105, -7.390897758835778930, 8.498862081921462419 ) ) ;
#8995=VERTEX_POINT ( 'NONE', #3321 ) ;
#8999=CARTESIAN_POINT ( 'NONE',  ( 9.837026868206066865, -5.012215536711391195, 10.35000000000002274 ) ) ;
#9005=CARTESIAN_POINT ( 'NONE',  ( 10.36326688006723984, -1.689666864740212215, 12.20113791807854398 ) ) ;
#9006=CARTESIAN_POINT ( 'NONE',  ( -9.377220287598998283, -4.724406229267462898, 4.401137918078569022 ) ) ;
#9012=CARTESIAN_POINT ( 'NONE',  ( 9.355568503977840678, 4.766900247265305701, 9.900000000000019895 ) ) ;
#9019=CARTESIAN_POINT ( 'NONE',  ( -8.486213763410637156, -4.270415729527911708, 1.401137918078568134 ) ) ;
#9020=CARTESIAN_POINT ( 'NONE',  ( -8.464561979789474222, -4.312909747525729642, 14.39999999999996838 ) ) ;
#9029=CARTESIAN_POINT ( 'NONE',  ( 6.751237864895159646, -6.683790977649239906, 20.49886208192143400 ) ) ;
#9030=CARTESIAN_POINT ( 'NONE',  ( 4.270415729527831772, 8.486213763410694000, 10.59886208192144075 ) ) ;
#9045=CARTESIAN_POINT ( 'NONE',  ( -10.89658364409024749, -1.776620879821561694, 3.548862081921419609 ) ) ;
#9054=CARTESIAN_POINT ( 'NONE',  ( 4.270415729527831772, 8.486213763410688671, 1.598862081921434308 ) ) ;
#9056=CARTESIAN_POINT ( 'NONE',  ( -1.727091770866549414, -10.90442828429184630, 1.949999999999996181 ) ) ;
#9057=CARTESIAN_POINT ( 'NONE',  ( 10.91227292449344155, 1.677562661911773167, 6.051137918078538291 ) ) ;
#9062=CARTESIAN_POINT ( 'NONE',  ( 9.837026868206066865, -5.012215536711391195, 4.350000000000036948 ) ) ;
#9068=CARTESIAN_POINT ( 'NONE',  ( 4.355403765523470305, 8.442910196168364578, 2.601137918078560762 ) ) ;
#9069=CARTESIAN_POINT ( 'NONE',  ( 7.063212654743467489, 7.063212654743553642, 15.74999999999996803 ) ) ;
#9079=CARTESIAN_POINT ( 'NONE',  ( 6.751237864895159646, -6.683790977649233689, 14.49886208192142867 ) ) ;
#9080=CARTESIAN_POINT ( 'NONE',  ( 7.027753727702739539, 7.098671581784288698, 7.748862081921418010 ) ) ;
#9095=CARTESIAN_POINT ( 'NONE',  ( -4.766900247265192014, -9.355568503977876205, 14.10000000000000142 ) ) ;
#9106=CARTESIAN_POINT ( 'NONE',  ( -7.771249796623103556, -7.842167650704634063, 18.24886208192143044 ) ) ;
#9108=CARTESIAN_POINT ( 'NONE',  ( -1.727091770866549414, -10.90442828429185695, 4.950000000000017053 ) ) ;
#9109=CARTESIAN_POINT ( 'NONE',  ( 4.967534682030706250, -9.859792900771036983, 6.651137918078563693 ) ) ;
#9114=CARTESIAN_POINT ( 'NONE',  ( 7.806708723663831506, 7.806708723663930982, 6.749999999999960032 ) ) ;
#9123=CARTESIAN_POINT ( 'NONE',  ( 1.439022436064387511, -9.390499931835510239, 15.80113791807855961 ) ) ;
#9124=CARTESIAN_POINT ( 'NONE',  ( -1.439022436064386845, 9.390499931835535108, -0.6988620819214501623 ) ) ;
#9136=CARTESIAN_POINT ( 'NONE',  ( 8.464561979789474222, 4.312909747525755400, 6.899999999999961275 ) ) ;
#9137=CARTESIAN_POINT ( 'NONE',  ( 1.533232399700100945, -9.375578539472073203, 11.79886208192143471 ) ) ;
#9138=CARTESIAN_POINT ( 'NONE',  ( -10.37072757624895836, 1.642561882922380034, 14.69999999999999041 ) ) ;
#9146=CARTESIAN_POINT ( 'NONE',  ( 7.806708723663831506, 7.806708723663925653, 15.74999999999996803 ) ) ;
#9150=CARTESIAN_POINT ( 'NONE',  ( -9.859792900771106261, 4.967534682030611215, 3.848862081921410105 ) ) ;
#9156=CARTESIAN_POINT ( 'NONE',  ( 9.355568503977840678, 4.766900247265305701, 18.90000000000002700 ) ) ;
#9159=CARTESIAN_POINT ( 'NONE',  ( -4.724406229267374968, -9.377220287599040915, 18.09886208192144252 ) ) ;
#9161=CARTESIAN_POINT ( 'NONE',  ( 5.012215536711511987, -9.837026868205999364, 1.650000000000006128 ) ) ;
#9162=CARTESIAN_POINT ( 'NONE',  ( 1.776620879821457333, 10.89658364409027236, 14.45113791807853509 ) ) ;
#9167=CARTESIAN_POINT ( 'NONE',  ( -10.37072757624895836, 1.642561882922381145, 5.700000000000038369 ) ) ;
#9173=CARTESIAN_POINT ( 'NONE',  ( 4.355403765523470305, 8.442910196168369907, 17.60113791807856742 ) ) ;
#9174=CARTESIAN_POINT ( 'NONE',  ( -9.383039235653820143, 1.486127417882154411, 11.69999999999998863 ) ) ;
#9184=CARTESIAN_POINT ( 'NONE',  ( -10.37072757624895836, 1.642561882922380923, 2.699999999999980194 ) ) ;
#9185=CARTESIAN_POINT ( 'NONE',  ( 4.312909747525650594, 8.464561979789541724, 6.599999999999994316 ) ) ;
#9186=CARTESIAN_POINT ( 'NONE',  ( -8.442910196168309511, -4.355403765523544024, 12.39886208192140948 ) ) ;
#9187=CARTESIAN_POINT ( 'NONE',  ( 10.37072757624895836, -1.642561882922355831, 19.19999999999999574 ) ) ;
#9195=CARTESIAN_POINT ( 'NONE',  ( 1.727091770866550968, 10.90442828429186761, 18.44999999999999218 ) ) ;
#9199=CARTESIAN_POINT ( 'NONE',  ( -7.806708723663830618, -7.806708723663902560, 14.25000000000001243 ) ) ;
#9209=CARTESIAN_POINT ( 'NONE',  ( 7.771249796623105333, 7.842167650704658932, 19.74886208192143044 ) ) ;
#9210=CARTESIAN_POINT ( 'NONE',  ( 7.806708723663831506, 7.806708723663925653, 9.749999999999982236 ) ) ;
#9211=CARTESIAN_POINT ( 'NONE',  ( -10.91227292449344155, -1.677562661911747632, 16.55113791807855605 ) ) ;
#9213=CARTESIAN_POINT ( 'NONE',  ( 4.766900247265192903, 9.355568503977902850, 15.60000000000000320 ) ) ;
#9215=CARTESIAN_POINT ( 'NONE',  ( -5.012215536711508435, 9.837026868206027785, 0.1499999999999952482 ) ) ;
#9218=CARTESIAN_POINT ( 'NONE',  ( 6.683790977649321619, -6.751237864895076157, 18.50113791807859087 ) ) ;
#9219=CARTESIAN_POINT ( 'NONE',  ( -1.439022436064386845, 9.390499931835526226, 2.301137918078551614 ) ) ;
#9230=CARTESIAN_POINT ( 'NONE',  ( -6.717514421272238856, 6.717514421272181124, 6.000000000000005329 ) ) ;
#9231=CARTESIAN_POINT ( 'NONE',  ( 8.922933199037192509, -4.490180821391404287, 14.34886208192142831 ) ) ;
#9232=CARTESIAN_POINT ( 'NONE',  ( -7.424621202458789426, 7.424621202458724589, 12.00000000000001066 ) ) ;
#9241=CARTESIAN_POINT ( 'NONE',  ( -1.727091770866549414, -10.90442828429184630, 13.95000000000002593 ) ) ;
#9246=CARTESIAN_POINT ( 'NONE',  ( 1.727091770866550968, 10.90442828429187294, 15.44999999999997797 ) ) ;
#9259=CARTESIAN_POINT ( 'NONE',  ( -7.458344646081709328, 7.390897758835805575, 18.99886208192142334 ) ) ;
#9261=CARTESIAN_POINT ( 'NONE',  ( -4.766900247265192014, -9.355568503977876205, 2.099999999999990763 ) ) ;
#9262=CARTESIAN_POINT ( 'NONE',  ( 9.814260835641038128, -5.056896391392198709, 18.35113791807858519 ) ) ;
#9270=CARTESIAN_POINT ( 'NONE',  ( 4.766900247265192903, 9.355568503977902850, 3.599999999999992095 ) ) ;
#9276=CARTESIAN_POINT ( 'NONE',  ( 10.36326688006723984, -1.689666864740212215, 0.2011379180785754783 ) ) ;
#9277=CARTESIAN_POINT ( 'NONE',  ( 9.873755945037075321, 1.513077731353043243, 9.051137918078573819 ) ) ;
#9290=CARTESIAN_POINT ( 'NONE',  ( 8.464561979789474222, 4.312909747525755400, 3.899999999999959055 ) ) ;
#9291=CARTESIAN_POINT ( 'NONE',  ( 1.533232399700100945, -9.375578539472067874, 17.79886208192143471 ) ) ;
#9302=CARTESIAN_POINT ( 'NONE',  ( -9.333916720356675967, -4.809394265263095214, 12.39886208192140948 ) ) ;
#9308=CARTESIAN_POINT ( 'NONE',  ( -1.486127417882243895, 9.383039235653825472, 6.299999999999972289 ) ) ;
#9314=CARTESIAN_POINT ( 'NONE',  ( 6.751237864895159646, -6.683790977649233689, 8.498862081921462419 ) ) ;
#9317=CARTESIAN_POINT ( 'NONE',  ( 10.91227292449344155, 1.677562661911773390, 15.05113791807855961 ) ) ;
#9327=CARTESIAN_POINT ( 'NONE',  ( -1.439022436064386845, 9.390499931835535108, 14.30113791807856316 ) ) ;
#9328=CARTESIAN_POINT ( 'NONE',  ( 8.877401133907127928, -4.579542530753017537, 3.351137918078579858 ) ) ;
#9339=CARTESIAN_POINT ( 'NONE',  ( 10.37072757624895836, -1.642561882922355831, 1.200000000000034373 ) ) ;
#9340=CARTESIAN_POINT ( 'NONE',  ( 4.312909747525650594, 8.464561979789532842, 3.599999999999992095 ) ) ;
#9341=CARTESIAN_POINT ( 'NONE',  ( 6.751237864895159646, -6.683790977649233689, 17.49886208192142689 ) ) ;
#9347=CARTESIAN_POINT ( 'NONE',  ( -9.355568503977838901, -4.766900247265279944, 11.39999999999996660 ) ) ;
#9351=CARTESIAN_POINT ( 'NONE',  ( 9.333916720356675967, 4.809394265263126300, 7.898862081921404155 ) ) ;
#9357=CARTESIAN_POINT ( 'NONE',  ( 4.534861676072321046, -8.900167166472098046, 10.65000000000001101 ) ) ;
#9363=CARTESIAN_POINT ( 'NONE',  ( 4.270415729527831772, 8.486213763410697553, 7.598862081921438971 ) ) ;
#9365=CARTESIAN_POINT ( 'NONE',  ( -1.727091770866549414, -10.90442828429184630, 1.949999999999996181 ) ) ;
#9366=CARTESIAN_POINT ( 'NONE',  ( -1.776620879821455556, -10.89658364409025637, 15.95113791807857595 ) ) ;
#9372=CARTESIAN_POINT ( 'NONE',  ( 9.837026868206070418, -5.012215536711392083, 7.350000000000000533 ) ) ;
#9376=CARTESIAN_POINT ( 'NONE',  ( 7.842167650704563897, 7.771249796623202144, 8.751137918078539357 ) ) ;
#9377=CARTESIAN_POINT ( 'NONE',  ( 7.098671581784200768, 7.027753727702831021, 5.751137918078548239 ) ) ;
#9386=MECHANICAL_DESIGN_GEOMETRIC_PRESENTATION_REPRESENTATION('',(#4756),#1279);
#9389=CARTESIAN_POINT ( 'NONE',  ( 6.683790977649321619, -6.751237864895077045, 0.5011379180785839882 ) ) ;
#9390=CARTESIAN_POINT ( 'NONE',  ( 7.063212654743467489, 7.063212654743557195, 0.7499999999999762412 ) ) ;
#9392=CARTESIAN_POINT ( 'NONE',  ( -9.383039235653820143, 1.486127417882155299, 2.700000000000035705 ) ) ;
#9402=CARTESIAN_POINT ( 'NONE',  ( 10.89658364409024749, 1.776620879821585897, 5.048862081921459577 ) ) ;
#9407=CARTESIAN_POINT ( 'NONE',  ( -8.464561979789474222, -4.312909747525728754, 11.39999999999996660 ) ) ;
#9408=CARTESIAN_POINT ( 'NONE',  ( -1.727091770866549414, -10.90442828429184630, 16.94999999999998863 ) ) ;
#9414=CARTESIAN_POINT ( 'NONE',  ( 4.270415729527831772, 8.486213763410688671, 13.59886208192144430 ) ) ;
#9418=CARTESIAN_POINT ( 'NONE',  ( 4.766900247265192903, 9.355568503977911732, 9.599999999999997868 ) ) ;
#9420=( LENGTH_UNIT ( ) NAMED_UNIT ( * ) SI_UNIT ( .MILLI., .METRE. ) );
#9427=CARTESIAN_POINT ( 'NONE',  ( 1.776620879821457333, 10.89658364409028124, 2.451137918078564848 ) ) ;
#9428=CARTESIAN_POINT ( 'NONE',  ( -4.490180821391513533, 8.922933199037158758, 17.15113791807853616 ) ) ;
#9445=CARTESIAN_POINT ( 'NONE',  ( 1.612135949262739398, 9.858066664633913234, -0.5488620819214271584 ) ) ;
#9446=CARTESIAN_POINT ( 'NONE',  ( -1.513077731352923339, -9.873755945037078874, 14.94886208192145105 ) ) ;
#9449=CARTESIAN_POINT ( 'NONE',  ( -4.534861676072319270, 8.900167166472122915, 3.149999999999958611 ) ) ;
#9455=CLOSED_SHELL ( 'NONE', ( #1076, #4264, #3959, #7548 ) ) ;
#9458=ADVANCED_BREP_SHAPE_REPRESENTATION ( '', ( #206, #3995 ), #6704 ) ;
#9459=CARTESIAN_POINT ( 'NONE',  ( 7.771249796623105333, 7.842167650704654491, 13.74886208192144643 ) ) ;
#9465=CARTESIAN_POINT ( 'NONE',  ( 4.534861676072321046, -8.900167166472098046, 13.65000000000003411 ) ) ;
#9466=CARTESIAN_POINT ( 'NONE',  ( 1.677562661911645714, 10.91227292449347175, 1.448862081921441947 ) ) ;
#9468=ORIENTED_EDGE ( 'NONE', *, *, #3511, .T. ) ;
#9469=DIRECTION ( 'NONE',  ( -0.7063021515967564667, -0.7063021515967625730, -0.04769215134145720486 ) ) ;
#9476=CARTESIAN_POINT ( 'NONE',  ( -4.766900247265192014, -9.355568503977876205, 5.099999999999993427 ) ) ;
#9481=CARTESIAN_POINT ( 'NONE',  ( -7.424621202458789426, 7.424621202458724589, 12.00000000000001066 ) ) ;
#9484=CARTESIAN_POINT ( 'NONE',  ( -4.809394265263009061, -9.333916720356716823, 7.101137918078564759 ) ) ;
#9485=CARTESIAN_POINT ( 'NONE',  ( 4.809394265263009061, 9.333916720356739916, -0.3988620819214416247 ) ) ;
#9494=CARTESIAN_POINT ( 'NONE',  ( -4.312909747525649706, -8.464561979789507973, 17.10000000000000497 ) ) ;
#9495=CARTESIAN_POINT ( 'NONE',  ( 4.312909747525650594, 8.464561979789532842, 3.599999999999992095 ) ) ;
#9507=CARTESIAN_POINT ( 'NONE',  ( 9.390499931835536884, -1.439022436064273158, 2.198862081921450606 ) ) ;
#9508=CARTESIAN_POINT ( 'NONE',  ( 7.771249796623105333, 7.842167650704658932, 7.748862081921418010 ) ) ;
#9513=CARTESIAN_POINT ( 'NONE',  ( -6.717514421272238856, 6.717514421272180236, 9.000000000000007105 ) ) ;
#9514=CARTESIAN_POINT ( 'NONE',  ( 1.689666864740335894, -10.36326688006721497, 2.798862081921426714 ) ) ;
#9521=CARTESIAN_POINT ( 'NONE',  ( 1.727091770866550968, 10.90442828429187294, 3.450000000000006839 ) ) ;
#9522=CARTESIAN_POINT ( 'NONE',  ( 10.37072757624895836, -1.642561882922355831, 1.200000000000034373 ) ) ;
#9527=CARTESIAN_POINT ( 'NONE',  ( -10.37072757624895836, 1.642561882922380923, 17.69999999999999218 ) ) ;
#9531=CARTESIAN_POINT ( 'NONE',  ( -4.809394265263009061, -9.333916720356718599, 1.101137918078559208 ) ) ;
#9532=CARTESIAN_POINT ( 'NONE',  ( 4.355403765523470305, 8.442910196168369907, 14.60113791807856920 ) ) ;
#9541=CARTESIAN_POINT ( 'NONE',  ( -1.439022436064386845, 9.390499931835535108, -0.6988620819214501623 ) ) ;
#9542=CARTESIAN_POINT ( 'NONE',  ( 4.312909747525650594, 8.464561979789541724, 9.599999999999997868 ) ) ;
#9545=CARTESIAN_POINT ( 'NONE',  ( 6.717514421272239744, -6.717514421272154479, 1.500000000000001332 ) ) ;
#9554=CARTESIAN_POINT ( 'NONE',  ( 5.056896391392317724, -9.814260835640977731, 14.64886208192141659 ) ) ;
#9555=CARTESIAN_POINT ( 'NONE',  ( 10.89658364409024749, 1.776620879821585897, 2.048862081921423162 ) ) ;
#9556=CARTESIAN_POINT ( 'NONE',  ( 10.89658364409024749, 1.776620879821587229, 14.04886208192143471 ) ) ;
#9563=CARTESIAN_POINT ( 'NONE',  ( 1.727091770866550968, 10.90442828429187294, 15.44999999999997797 ) ) ;
#9570=CARTESIAN_POINT ( 'NONE',  ( -10.37072757624895836, 1.642561882922380034, 11.69999999999998863 ) ) ;
#9571=CARTESIAN_POINT ( 'NONE',  ( 1.727091770866550968, 10.90442828429187294, 0.4499999999999856337 ) ) ;
#9573=PRESENTATION_STYLE_ASSIGNMENT (( #891 ) ) ;
#9576=CARTESIAN_POINT ( 'NONE',  ( -7.806708723663831506, -7.806708723663903449, 14.25000000000001421 ) ) ;
#9579=CARTESIAN_POINT ( 'NONE',  ( 4.809394265263009061, 9.333916720356739916, 5.601137918078562983 ) ) ;
#9580=CARTESIAN_POINT ( 'NONE',  ( -8.486213763410637156, -4.270415729527911708, 10.40113791807857524 ) ) ;
#9592=CIRCLE ( 'NONE', #4792, 0.4999999999999994449 ) ;
#9593=CARTESIAN_POINT ( 'NONE',  ( -9.865911304835474738, -1.562606840307925626, 14.55000000000000249 ) ) ;
#9594=CARTESIAN_POINT ( 'NONE',  ( -1.486127417882243895, 9.383039235653825472, 6.299999999999972289 ) ) ;
#9595=DIRECTION ( 'NONE',  ( 0.7063021515967569108, 0.7063021515967621289, -0.04769215134145721874 ) ) ;
#9609=CARTESIAN_POINT ( 'NONE',  ( 4.270415729527831772, 8.486213763410694000, 10.59886208192144075 ) ) ;
#9610=CARTESIAN_POINT ( 'NONE',  ( 7.771249796623105333, 7.842167650704658932, 19.74886208192143044 ) ) ;
#9618=CARTESIAN_POINT ( 'NONE',  ( 7.063212654743468377, 7.063212654743559860, 18.74999999999998934 ) ) ;
#9619=CARTESIAN_POINT ( 'NONE',  ( -9.859792900771106261, 4.967534682030611215, 3.848862081921410105 ) ) ;
#9626=CARTESIAN_POINT ( 'NONE',  ( 10.37072757624895836, -1.642561882922356498, 13.19999999999998863 ) ) ;
#9627=CARTESIAN_POINT ( 'NONE',  ( 5.012215536711511987, -9.837026868205997587, 7.649999999999992362 ) ) ;
#9631=CARTESIAN_POINT ( 'NONE',  ( -4.766900247265192014, -9.355568503977867323, 11.09999999999999787 ) ) ;
#9635=CARTESIAN_POINT ( 'NONE',  ( -1.595456901104623348, 10.37818827243066622, 11.30113791807855961 ) ) ;
#9636=CARTESIAN_POINT ( 'NONE',  ( -8.486213763410637156, -4.270415729527911708, 13.40113791807857702 ) ) ;
#9646=CARTESIAN_POINT ( 'NONE',  ( 9.375578539472099848, -1.533232399699986370, 9.201137918078538647 ) ) ;
#9647=CARTESIAN_POINT ( 'NONE',  ( -1.562606840307830591, -9.865911304835478290, 1.949999999999996181 ) ) ;
#9658=CARTESIAN_POINT ( 'NONE',  ( -1.677562661911643938, -10.91227292449344688, 14.94886208192145105 ) ) ;
#9664=CARTESIAN_POINT ( 'NONE',  ( 1.562606840307832146, 9.865911304835501383, 18.44999999999999929 ) ) ;
#9665=CARTESIAN_POINT ( 'NONE',  ( -9.859792900771106261, 4.967534682030606774, 6.848862081921402556 ) ) ;
#9672=CARTESIAN_POINT ( 'NONE',  ( 1.727091770866550968, 10.90442828429187294, 9.449999999999988631 ) ) ;
#9673=CARTESIAN_POINT ( 'NONE',  ( 7.424621202458790314, -7.424621202458697944, 10.50000000000000888 ) ) ;
#9677=CARTESIAN_POINT ( 'NONE',  ( 9.355568503977840678, 4.766900247265305701, 15.90000000000002522 ) ) ;
#9681=CARTESIAN_POINT ( 'NONE',  ( -9.377220287598998283, -4.724406229267462898, 10.40113791807857524 ) ) ;
#9682=CARTESIAN_POINT ( 'NONE',  ( -7.842167650704559456, -7.771249796623176387, 1.251137918078559563 ) ) ;
#9690=CARTESIAN_POINT ( 'NONE',  ( -8.486213763410637156, -4.270415729527911708, 4.401137918078569022 ) ) ;
#9691=CARTESIAN_POINT ( 'NONE',  ( 1.486127417882244783, -9.383039235653791721, 1.800000000000023803 ) ) ;
#9702=CARTESIAN_POINT ( 'NONE',  ( 7.027753727702739539, 7.098671581784283369, 13.74886208192144643 ) ) ;
#9703=CARTESIAN_POINT ( 'NONE',  ( 5.056896391392317724, -9.814260835640970626, 17.64886208192141126 ) ) ;
#9713=CARTESIAN_POINT ( 'NONE',  ( 9.859792900771104485, -4.967534682030585458, 5.348862081921449629 ) ) ;
#9720=CARTESIAN_POINT ( 'NONE',  ( -1.727091770866549414, -10.90442828429184630, 10.95000000000000462 ) ) ;
#9721=CARTESIAN_POINT ( 'NONE',  ( 9.355568503977840678, 4.766900247265305701, 18.90000000000002700 ) ) ;
#9727=CARTESIAN_POINT ( 'NONE',  ( 7.806708723663832394, 7.806708723663931870, 18.74999999999998934 ) ) ;
#9732=CARTESIAN_POINT ( 'NONE',  ( -1.642561882922479732, 10.37072757624895303, 0.2999999999999669598 ) ) ;
#9733=CARTESIAN_POINT ( 'NONE',  ( -10.91227292449344155, -1.677562661911747632, 1.551137918078593803 ) ) ;
#9737=CARTESIAN_POINT ( 'NONE',  ( 5.012215536711511987, -9.837026868205999364, 10.65000000000000924 ) ) ;
#9742=CARTESIAN_POINT ( 'NONE',  ( 4.312909747525650594, 8.464561979789532842, 18.60000000000000497 ) ) ;
#9751=CARTESIAN_POINT ( 'NONE',  ( 7.071067811865515473, -7.071067811865425767, 19.50000000000001776 ) ) ;
#9755=CARTESIAN_POINT ( 'NONE',  ( -6.751237864895158758, 6.683790977649261222, 18.99886208192142334 ) ) ;
#9756=CARTESIAN_POINT ( 'NONE',  ( -7.027753727702738651, -7.098671581784262941, 6.248862081921465084 ) ) ;
#9766=CARTESIAN_POINT ( 'NONE',  ( -10.89658364409024749, -1.776620879821561694, 3.548862081921419609 ) ) ;
#9773=CARTESIAN_POINT ( 'NONE',  ( 7.806708723663831506, 7.806708723663925653, 9.749999999999982236 ) ) ;
#9785=CARTESIAN_POINT ( 'NONE',  ( -9.377220287598998283, -4.724406229267462898, 13.40113791807857702 ) ) ;
#9786=CARTESIAN_POINT ( 'NONE',  ( 1.776620879821457333, 10.89658364409028124, 5.451137918078557298 ) ) ;
#9790=CARTESIAN_POINT ( 'NONE',  ( 10.90442828429183919, 1.727091770866679310, 7.050000000000010481 ) ) ;
#9796=CARTESIAN_POINT ( 'NONE',  ( -8.877401133907129704, 4.579542530753039742, 1.851137918078540334 ) ) ;
#9797=CARTESIAN_POINT ( 'NONE',  ( -9.865911304835474738, -1.562606840307925626, 17.55000000000002913 ) ) ;
#9805=PRODUCT ( 'small spring', 'small spring', '', ( #2009 ) ) ;
#9807=CARTESIAN_POINT ( 'NONE',  ( -1.533232399700100057, 9.375578539472098072, 16.29886208192143471 ) ) ;
#9808=CARTESIAN_POINT ( 'NONE',  ( -1.513077731352923339, -9.873755945037078874, 8.948862081921467038 ) ) ;
#9816=CARTESIAN_POINT ( 'NONE',  ( -5.056896391392315948, 9.814260835640991942, 4.148862081921444123 ) ) ;
#9822=CARTESIAN_POINT ( 'NONE',  ( 10.90442828429183919, 1.727091770866679532, 16.04999999999995808 ) ) ;
#9830=CARTESIAN_POINT ( 'NONE',  ( -9.390499931835536884, 1.439022436064298249, 3.698862081921452827 ) ) ;
#9832=CARTESIAN_POINT ( 'NONE',  ( -10.91227292449344155, -1.677562661911747632, 16.55113791807855605 ) ) ;
#9833=CARTESIAN_POINT ( 'NONE',  ( 9.377220287599001836, 4.724406229267489543, 5.901137918078571687 ) ) ;
#9835=CARTESIAN_POINT ( 'NONE',  ( -1.642561882922479732, 10.37072757624896191, 6.299999999999972289 ) ) ;
#9841=CARTESIAN_POINT ( 'NONE',  ( -7.098671581784199880, -7.027753727702809705, 4.251137918078595312 ) ) ;
#9842=CARTESIAN_POINT ( 'NONE',  ( -7.063212654743466601, -7.063212654743531438, 11.24999999999999467 ) ) ;
#9852=CARTESIAN_POINT ( 'NONE',  ( -6.751237864895158758, 6.683790977649261222, 15.99886208192142512 ) ) ;
#9853=CARTESIAN_POINT ( 'NONE',  ( -9.390499931835536884, 1.439022436064298249, 6.698862081921455491 ) ) ;
#9867=CARTESIAN_POINT ( 'NONE',  ( 9.837026868206066865, -5.012215536711392083, 13.34999999999998188 ) ) ;
#9874=CARTESIAN_POINT ( 'NONE',  ( 1.727091770866551412, 10.90442828429186761, 18.44999999999999929 ) ) ;
#9876=CARTESIAN_POINT ( 'NONE',  ( 10.37818827243067510, -1.595456901104500780, 17.19886208192146171 ) ) ;
#9878=CARTESIAN_POINT ( 'NONE',  ( -7.806708723663830618, -7.806708723663906113, 2.249999999999986233 ) ) ;
#9879=CARTESIAN_POINT ( 'NONE',  ( 7.842167650704563897, 7.771249796623202144, 5.751137918078548239 ) ) ;
#9884=CARTESIAN_POINT ( 'NONE',  ( -1.727091770866549414, -10.90442828429184630, 10.95000000000000462 ) ) ;
#9890=CARTESIAN_POINT ( 'NONE',  ( -4.490180821391513533, 8.922933199037153429, 14.15113791807854327 ) ) ;
#9891=CARTESIAN_POINT ( 'NONE',  ( 8.900167166472154889, -4.534861676072213577, 16.35000000000000497 ) ) ;
#9903=CARTESIAN_POINT ( 'NONE',  ( 4.312909747525650594, 8.464561979789532842, 0.5999999999999894307 ) ) ;
#9904=CARTESIAN_POINT ( 'NONE',  ( -7.027753727702738651, -7.098671581784268270, 3.248862081921429112 ) ) ;
#9906=CARTESIAN_POINT ( 'NONE',  ( 4.766900247265192903, 9.355568503977902850, 15.60000000000000320 ) ) ;
#9924=CARTESIAN_POINT ( 'NONE',  ( -7.771249796623103556, -7.842167650704637616, 3.248862081921429112 ) ) ;
#9932=CARTESIAN_POINT ( 'NONE',  ( 4.724406229267374968, 9.377220287599060455, 19.59886208192140700 ) ) ;
#9935=CARTESIAN_POINT ( 'NONE',  ( -9.355568503977838901, -4.766900247265280832, 8.399999999999963052 ) ) ;
#9936=CARTESIAN_POINT ( 'NONE',  ( -7.842167650704559456, -7.771249796623176387, 10.25113791807858021 ) ) ;
#9938=CARTESIAN_POINT ( 'NONE',  ( -5.012215536711506658, 9.837026868206027785, 9.150000000000003908 ) ) ;
#9944=CARTESIAN_POINT ( 'NONE',  ( 1.612135949262739398, 9.858066664633906129, 14.45113791807853509 ) ) ;
#9945=CARTESIAN_POINT ( 'NONE',  ( -4.312909747525649706, -8.464561979789507973, 14.10000000000000142 ) ) ;
#9958=CARTESIAN_POINT ( 'NONE',  ( -8.464561979789474222, -4.312909747525728754, 5.400000000000016342 ) ) ;
#9959=CARTESIAN_POINT ( 'NONE',  ( 7.027753727702739539, 7.098671581784288698, 10.74886208192140913 ) ) ;
#9960=CARTESIAN_POINT ( 'NONE',  ( -7.806708723663830618, -7.806708723663901672, 11.24999999999999467 ) ) ;
#9966=CARTESIAN_POINT ( 'NONE',  ( 1.727091770866550968, 10.90442828429187294, 15.44999999999997797 ) ) ;
#9970=CARTESIAN_POINT ( 'NONE',  ( -7.424621202458789426, 7.424621202458723701, 15.00000000000001421 ) ) ;
#9980=CARTESIAN_POINT ( 'NONE',  ( 8.922933199037192509, -4.490180821391404287, 5.348862081921449629 ) ) ;
#9982=CARTESIAN_POINT ( 'NONE',  ( -1.642561882922479732, 10.37072757624896191, 9.299999999999975842 ) ) ;
#9983=CARTESIAN_POINT ( 'NONE',  ( -4.809394265263009061, -9.333916720356716823, 16.10113791807856742 ) ) ;
#9987=CARTESIAN_POINT ( 'NONE',  ( 1.642561882922480621, -10.37072757624892638, 13.80000000000003446 ) ) ;
#9992=CARTESIAN_POINT ( 'NONE',  ( 1.612135949262739398, 9.858066664633913234, 17.45113791807857240 ) ) ;
#9993=CARTESIAN_POINT ( 'NONE',  ( -6.683790977649319842, 6.751237864895101026, 8.001137918078546463 ) ) ;
#10003=CARTESIAN_POINT ( 'NONE',  ( 4.534861676072320158, -8.900167166472098046, 10.65000000000000924 ) ) ;
#10004=CARTESIAN_POINT ( 'NONE',  ( -4.270415729527831772, -8.486213763410670907, 15.09886208192144430 ) ) ;
#10005=CARTESIAN_POINT ( 'NONE',  ( -9.837026868206066865, 5.012215536711416064, 17.85000000000001918 ) ) ;
#10012=CARTESIAN_POINT ( 'NONE',  ( -1.727091770866549414, -10.90442828429184630, 10.95000000000000462 ) ) ;
#10016=CARTESIAN_POINT ( 'NONE',  ( 1.677562661911645714, 10.91227292449347175, 1.448862081921441947 ) ) ;
#10029=CARTESIAN_POINT ( 'NONE',  ( 7.027753727702739539, 7.098671581784288698, 1.748862081921432887 ) ) ;
#10031=CARTESIAN_POINT ( 'NONE',  ( -9.814260835641038128, 5.056896391392221801, 13.85113791807855321 ) ) ;
#10036=CARTESIAN_POINT ( 'NONE',  ( 1.727091770866551412, 10.90442828429187117, 0.4499999999999857447 ) ) ;
#10039=CARTESIAN_POINT ( 'NONE',  ( 9.873755945037075321, 1.513077731353044131, 12.05113791807856671 ) ) ;
#10040=CARTESIAN_POINT ( 'NONE',  ( 6.683790977649321619, -6.751237864895076157, 6.501137918078588207 ) ) ;
#10051=CARTESIAN_POINT ( 'NONE',  ( 7.806708723663831506, 7.806708723663930982, 0.7499999999999762412 ) ) ;
#10052=CARTESIAN_POINT ( 'NONE',  ( -7.063212654743466601, -7.063212654743531438, 11.24999999999999467 ) ) ;
#10053=CARTESIAN_POINT ( 'NONE',  ( 4.579542530753127672, -8.877401133907065756, 17.64886208192141126 ) ) ;
#10062=CARTESIAN_POINT ( 'NONE',  ( -1.642561882922479732, 10.37072757624895303, 18.29999999999998295 ) ) ;
#10065=CARTESIAN_POINT ( 'NONE',  ( 4.724406229267374968, 9.377220287599055126, 4.598862081921435419 ) ) ;
#10071=CARTESIAN_POINT ( 'NONE',  ( -4.312909747525649706, -8.464561979789499091, 8.099999999999996092 ) ) ;
#10079=CARTESIAN_POINT ( 'NONE',  ( -9.858066664633883036, -1.612135949262833101, 12.54886208192144004 ) ) ;
#10081=CARTESIAN_POINT ( 'NONE',  ( 9.837026868206066865, -5.012215536711392083, 7.350000000000000533 ) ) ;
#10082=CARTESIAN_POINT ( 'NONE',  ( -10.91227292449344155, -1.677562661911749187, 13.55113791807856316 ) ) ;
#10090=CARTESIAN_POINT ( 'NONE',  ( 9.355568503977840678, 4.766900247265305701, 3.899999999999959055 ) ) ;
#10096=CARTESIAN_POINT ( 'NONE',  ( -1.612135949262737844, -9.858066664633888365, 15.95113791807857595 ) ) ;
#10097=CARTESIAN_POINT ( 'NONE',  ( -7.098671581784199880, -7.027753727702804376, 1.251137918078559563 ) ) ;
#10109=CARTESIAN_POINT ( 'NONE',  ( 9.383039235653818366, -1.486127417882129986, 4.199999999999981526 ) ) ;
#10110=CARTESIAN_POINT ( 'NONE',  ( -8.922933199037192509, 4.490180821391428267, 12.84886208192143009 ) ) ;
#10116=CARTESIAN_POINT ( 'NONE',  ( -1.642561882922479732, 10.37072757624895303, 15.29999999999997939 ) ) ;
#10119=CARTESIAN_POINT ( 'NONE',  ( -7.458344646081709328, 7.390897758835799358, 12.99886208192142512 ) ) ;
#10123=CARTESIAN_POINT ( 'NONE',  ( -1.562606840307830591, -9.865911304835480067, 7.950000000000040146 ) ) ;
#10130=CARTESIAN_POINT ( 'NONE',  ( -4.270415729527831772, -8.486213763410678013, 12.09886208192144252 ) ) ;
#10133=CARTESIAN_POINT ( 'NONE',  ( -4.967534682030703586, 9.859792900771061852, 11.15113791807855215 ) ) ;
#10136=( NAMED_UNIT ( * ) PLANE_ANGLE_UNIT ( ) SI_UNIT ( $, .RADIAN. ) );
#10139=CARTESIAN_POINT ( 'NONE',  ( -10.37072757624895836, 1.642561882922381145, 5.700000000000038369 ) ) ;
#10143=CARTESIAN_POINT ( 'NONE',  ( 9.377220287599001836, 4.724406229267489543, 8.901137918078571687 ) ) ;
#10145=CARTESIAN_POINT ( 'NONE',  ( -8.486213763410637156, -4.270415729527911708, 4.401137918078569022 ) ) ;
#10156=CARTESIAN_POINT ( 'NONE',  ( 4.534861676072320158, -8.900167166472098046, 4.650000000000026112 ) ) ;
#10157=CARTESIAN_POINT ( 'NONE',  ( -1.486127417882243895, 9.383039235653816590, 0.2999999999999669598 ) ) ;
#10164=PRODUCT_DEFINITION ( 'UNKNOWN', '', #4436, #1123 ) ;
#10167=CARTESIAN_POINT ( 'NONE',  ( 4.724406229267374968, 9.377220287599055126, 13.59886208192140167 ) ) ;
#10173=CARTESIAN_POINT ( 'NONE',  ( -4.534861676072319270, 8.900167166472124691, 9.150000000000002132 ) ) ;
#10174=CARTESIAN_POINT ( 'NONE',  ( 9.837026868206066865, -5.012215536711395636, 16.35000000000000497 ) ) ;
#10181=CARTESIAN_POINT ( 'NONE',  ( 8.442910196168311288, 4.355403765523574222, 10.89886208192140771 ) ) ;
#10184=CARTESIAN_POINT ( 'NONE',  ( -9.355568503977838901, -4.766900247265280832, 8.399999999999963052 ) ) ;
#10195=CARTESIAN_POINT ( 'NONE',  ( 4.809394265263009061, 9.333916720356734587, 2.601137918078560762 ) ) ;
#10196=CARTESIAN_POINT ( 'NONE',  ( -8.486213763410637156, -4.270415729527909043, 7.401137918078573463 ) ) ;
#10206=CARTESIAN_POINT ( 'NONE',  ( 4.312909747525650594, 8.464561979789532842, 18.60000000000000497 ) ) ;
#10207=CARTESIAN_POINT ( 'NONE',  ( 1.513077731352925115, 9.873755945037103743, 16.44886208192140131 ) ) ;
#10220=CARTESIAN_POINT ( 'NONE',  ( -1.677562661911643938, -10.91227292449344688, 8.948862081921467038 ) ) ;
#10226=CARTESIAN_POINT ( 'NONE',  ( 8.900167166472158442, -4.534861676072210912, 13.34999999999998543 ) ) ;
ENDSEC;
END-ISO-10303-21;
